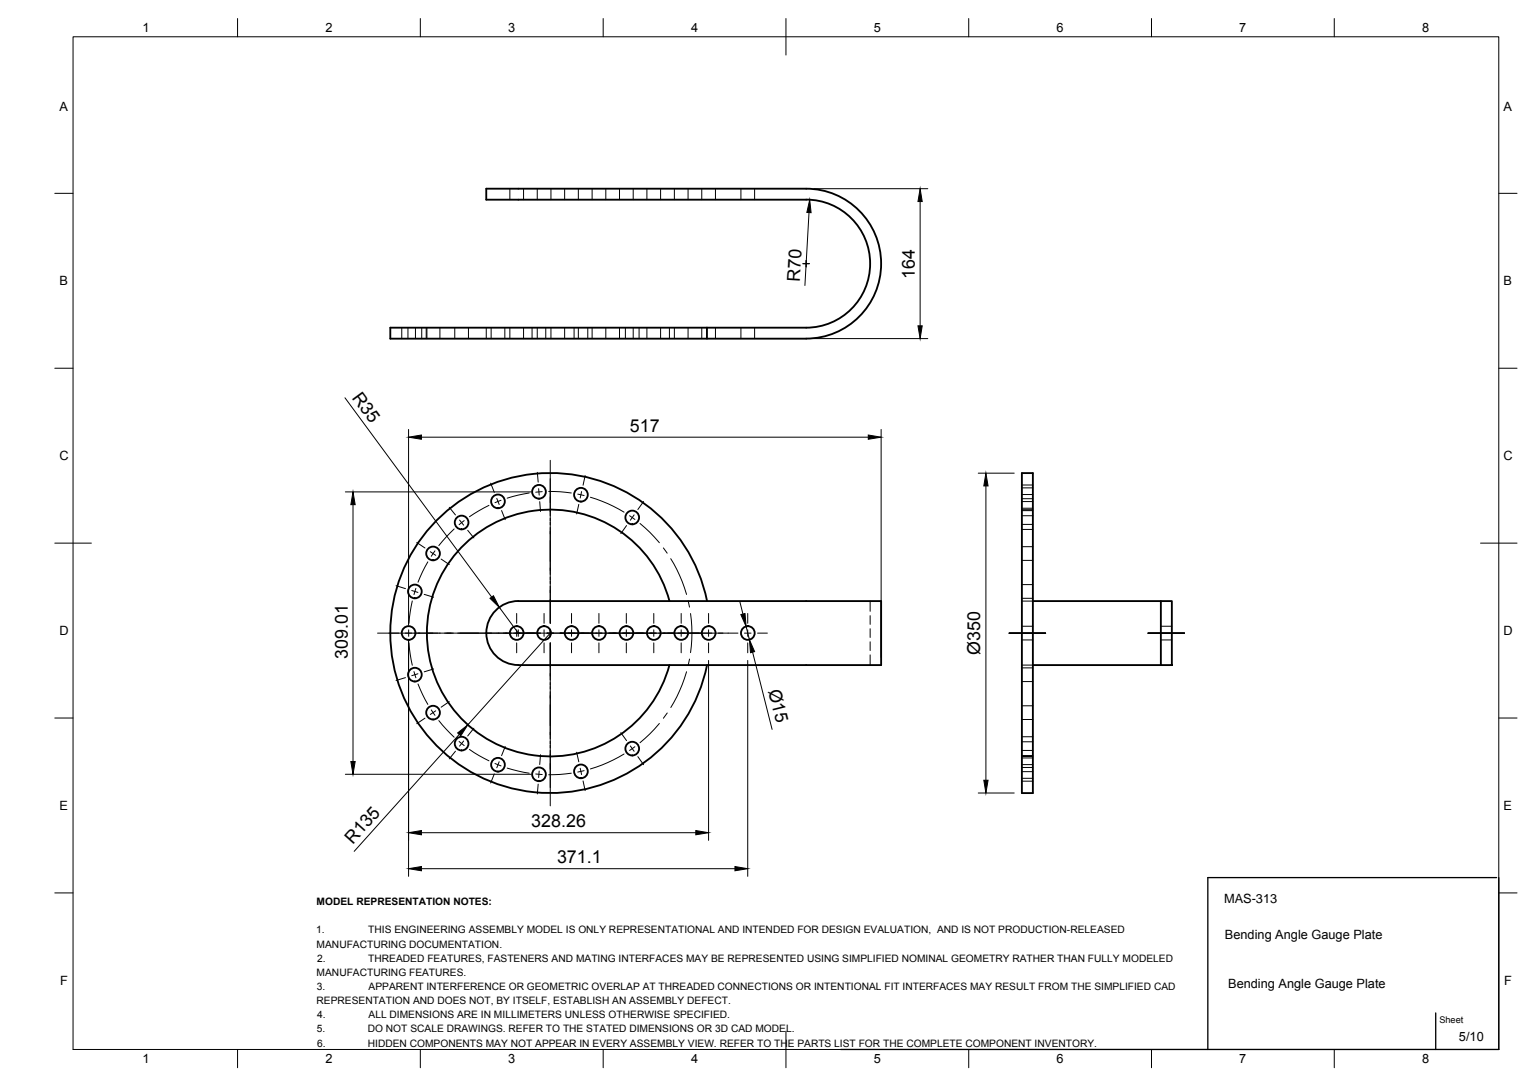
ISO-10303-21;
HEADER;
FILE_DESCRIPTION (('STEP AP214'),
    '1' );
FILE_NAME ('Bending Angle Gauge Plate.step',
    '2026-10-06T09:36:00',
    ( '' ),
    ( '' ),
    'SwSTEP 2.0',
    'SolidWorks 2025',
    '' );
FILE_SCHEMA (( 'AUTOMOTIVE_DESIGN' ));
ENDSEC;

DATA;
#1=ORIENTED_EDGE ( 'NONE', *, *, #10134, .F. ) ;
#14=EDGE_CURVE ( 'NONE', #10023, #7883, #9995, .T. ) ;
#18=CIRCLE ( 'NONE', #8899, 134.9999999999999716 ) ;
#26=DIRECTION ( 'NONE',  ( 0.000000000000000000, 0.000000000000000000, 1.000000000000000000 ) ) ;
#33=EDGE_CURVE ( 'NONE', #7221, #5849, #1766, .T. ) ;
#34=ORIENTED_EDGE ( 'NONE', *, *, #7230, .T. ) ;
#37=ORIENTED_EDGE ( 'NONE', *, *, #6606, .T. ) ;
#45=ORIENTED_EDGE ( 'NONE', *, *, #10615, .T. ) ;
#49=LINE ( 'NONE', #8712, #562 ) ;
#54=DIRECTION ( 'NONE',  ( -0.000000000000000000, 1.000000000000000000, 7.930164461608263644E-17 ) ) ;
#55=ORIENTED_EDGE ( 'NONE', *, *, #5184, .F. ) ;
#56=CARTESIAN_POINT ( 'NONE',  ( 1.561981751485805177E-12, 12.00000000000000000, 23.57864376269050410 ) ) ;
#62=FACE_BOUND ( 'NONE', #10137, .T. ) ;
#63=ORIENTED_EDGE ( 'NONE', *, *, #11154, .T. ) ;
#64=VERTEX_POINT ( 'NONE', #2451 ) ;
#74=AXIS2_PLACEMENT_3D ( 'NONE', #9091, #4403, #8176 ) ;
#75=EDGE_LOOP ( 'NONE', ( #6909, #2744, #1662, #2481 ) ) ;
#77=DIRECTION ( 'NONE',  ( 0.000000000000000000, 0.000000000000000000, 1.000000000000000000 ) ) ;
#83=VERTEX_POINT ( 'NONE', #3428 ) ;
#85=ORIENTED_EDGE ( 'NONE', *, *, #1558, .T. ) ;
#94=CYLINDRICAL_SURFACE ( 'NONE', #4643, 70.00000000000002842 ) ;
#97=AXIS2_PLACEMENT_3D ( 'NONE', #11633, #3261, #1306 ) ;
#101=ORIENTED_EDGE ( 'NONE', *, *, #4439, .T. ) ;
#110=ORIENTED_EDGE ( 'NONE', *, *, #8930, .F. ) ;
#115=DIRECTION ( 'NONE',  ( 0.000000000000000000, 1.000000000000000000, 0.000000000000000000 ) ) ;
#116=ORIENTED_EDGE ( 'NONE', *, *, #6003, .T. ) ;
#117=CYLINDRICAL_SURFACE ( 'NONE', #9034, 7.500000000000007105 ) ;
#122=ORIENTED_EDGE ( 'NONE', *, *, #10751, .T. ) ;
#123=FACE_BOUND ( 'NONE', #7167, .T. ) ;
#125=VERTEX_POINT ( 'NONE', #4313 ) ;
#131=CARTESIAN_POINT ( 'NONE',  ( -120.8820948793972434, 12.00000000000000000, -179.1989091883324363 ) ) ;
#133=VECTOR ( 'NONE', #10097, 1000.000000000000000 ) ;
#134=CARTESIAN_POINT ( 'NONE',  ( 1.387778780781445676E-14, -58.00000000000000711, 126.4213562373094959 ) ) ;
#135=ORIENTED_EDGE ( 'NONE', *, *, #8137, .F. ) ;
#148=DIRECTION ( 'NONE',  ( 0.000000000000000000, 0.000000000000000000, -1.000000000000000000 ) ) ;
#157=FACE_OUTER_BOUND ( 'NONE', #4978, .T. ) ;
#168=CYLINDRICAL_SURFACE ( 'NONE', #6692, 7.500000000000007105 ) ;
#173=ORIENTED_EDGE ( 'NONE', *, *, #11290, .T. ) ;
#175=VECTOR ( 'NONE', #6548, 1000.000000000000000 ) ;
#177=FACE_BOUND ( 'NONE', #6264, .T. ) ;
#184=ADVANCED_FACE ( 'NONE', ( #596 ), #4371, .T. ) ;
#186=CARTESIAN_POINT ( 'NONE',  ( 1.874378101782966050E-12, -6.000000000000006217, 61.07864376269051121 ) ) ;
#189=ORIENTED_EDGE ( 'NONE', *, *, #1792, .T. ) ;
#193=ORIENTED_EDGE ( 'NONE', *, *, #8592, .F. ) ;
#199=EDGE_CURVE ( 'NONE', #11915, #1856, #8826, .T. ) ;
#201=ORIENTED_EDGE ( 'NONE', *, *, #5756, .F. ) ;
#208=DIRECTION ( 'NONE',  ( -0.000000000000000000, 1.000000000000000000, 7.930164461608263644E-17 ) ) ;
#215=DIRECTION ( 'NONE',  ( -0.000000000000000000, 1.000000000000000000, 7.930164461608263644E-17 ) ) ;
#216=DIRECTION ( 'NONE',  ( 0.000000000000000000, 0.000000000000000000, 1.000000000000000000 ) ) ;
#217=ORIENTED_EDGE ( 'NONE', *, *, #11458, .T. ) ;
#224=LINE ( 'NONE', #2033, #3608 ) ;
#226=CYLINDRICAL_SURFACE ( 'NONE', #5194, 7.500000000000007105 ) ;
#231=CARTESIAN_POINT ( 'NONE',  ( 120.8820948793965186, 0.000000000000000000, -194.1989091883332890 ) ) ;
#235=EDGE_CURVE ( 'NONE', #11998, #11124, #7336, .T. ) ;
#239=CARTESIAN_POINT ( 'NONE',  ( 0.000000000000000000, 0.000000000000000000, -89.68077099980401101 ) ) ;
#241=ORIENTED_EDGE ( 'NONE', *, *, #8867, .F. ) ;
#242=CIRCLE ( 'NONE', #10114, 7.500000000000020428 ) ;
#244=CARTESIAN_POINT ( 'NONE',  ( 3.123963502971610252E-13, 12.00000000000000000, -96.42135623730949590 ) ) ;
#249=AXIS2_PLACEMENT_3D ( 'NONE', #6784, #11489, #10438 ) ;
#253=EDGE_CURVE ( 'NONE', #7231, #4288, #5520, .T. ) ;
#254=FACE_OUTER_BOUND ( 'NONE', #3985, .T. ) ;
#268=CARTESIAN_POINT ( 'NONE',  ( -35.00000000000000000, 81.99999999999998579, 190.3192290001959748 ) ) ;
#271=ADVANCED_FACE ( 'NONE', ( #9188 ), #1781, .F. ) ;
#277=ORIENTED_EDGE ( 'NONE', *, *, #5385, .T. ) ;
#278=CIRCLE ( 'NONE', #3844, 7.500000000000013323 ) ;
#281=ORIENTED_EDGE ( 'NONE', *, *, #1146, .T. ) ;
#285=CARTESIAN_POINT ( 'NONE',  ( -6.106226635438360972E-13, 0.000000000000000000, -244.6807709998039400 ) ) ;
#287=CIRCLE ( 'NONE', #5208, 7.500000000000007105 ) ;
#298=ORIENTED_EDGE ( 'NONE', *, *, #7352, .T. ) ;
#299=CARTESIAN_POINT ( 'NONE',  ( 3.123963502971610252E-13, 164.0000000000000000, -96.42135623730948168 ) ) ;
#315=ORIENTED_EDGE ( 'NONE', *, *, #3330, .T. ) ;
#319=CARTESIAN_POINT ( 'NONE',  ( 45.53315400109643463, 12.00000000000000000, -230.3419396193597208 ) ) ;
#321=EDGE_CURVE ( 'NONE', #10730, #10836, #6230, .T. ) ;
#328=EDGE_LOOP ( 'NONE', ( #135, #8709, #7075, #7838 ) ) ;
#333=DIRECTION ( 'NONE',  ( 0.000000000000000000, -1.156482317317870246E-16, 1.000000000000000000 ) ) ;
#338=VERTEX_POINT ( 'NONE', #2508 ) ;
#344=EDGE_LOOP ( 'NONE', ( #2553, #10547, #8461, #7126 ) ) ;
#348=CARTESIAN_POINT ( 'NONE',  ( 154.5043356068769071, 12.00000000000000000, -109.5666613060171670 ) ) ;
#350=CARTESIAN_POINT ( 'NONE',  ( 151.3258811035896656, 12.00000000000000000, -48.63263083939796871 ) ) ;
#356=DIRECTION ( 'NONE',  ( 0.000000000000000000, -1.000000000000000000, -7.930164461608263644E-17 ) ) ;
#362=AXIS2_PLACEMENT_3D ( 'NONE', #5126, #8886, #3258 ) ;
#367=CIRCLE ( 'NONE', #4729, 7.500000000000007105 ) ;
#371=CIRCLE ( 'NONE', #8725, 7.500000000000007105 ) ;
#383=EDGE_LOOP ( 'NONE', ( #2203, #8907 ) ) ;
#384=CARTESIAN_POINT ( 'NONE',  ( -151.3258811035894098, 12.00000000000000000, -48.63263083939678921 ) ) ;
#386=ORIENTED_EDGE ( 'NONE', *, *, #9875, .T. ) ;
#394=CYLINDRICAL_SURFACE ( 'NONE', #10869, 134.9999999999999716 ) ;
#403=EDGE_CURVE ( 'NONE', #4980, #6173, #8091, .T. ) ;
#404=FACE_BOUND ( 'NONE', #5340, .T. ) ;
#409=CARTESIAN_POINT ( 'NONE',  ( 1.874378101782966050E-12, 152.0000000000000000, 53.57864376269051832 ) ) ;
#411=DIRECTION ( 'NONE',  ( -0.000000000000000000, -1.000000000000000000, -0.000000000000000000 ) ) ;
#420=DIRECTION ( 'NONE',  ( -0.000000000000000000, 1.000000000000000000, 0.000000000000000000 ) ) ;
#421=DIRECTION ( 'NONE',  ( 0.000000000000000000, -1.189524669241239115E-16, 1.000000000000000000 ) ) ;
#422=LINE ( 'NONE', #11515, #6475 ) ;
#424=EDGE_LOOP ( 'NONE', ( #6274, #101, #7246, #3774 ) ) ;
#428=ORIENTED_EDGE ( 'NONE', *, *, #8066, .T. ) ;
#431=DIRECTION ( 'NONE',  ( 0.000000000000000000, 0.000000000000000000, 1.000000000000000000 ) ) ;
#435=ORIENTED_EDGE ( 'NONE', *, *, #33, .T. ) ;
#444=CARTESIAN_POINT ( 'NONE',  ( -35.00000000000000000, 12.00000000000000000, 81.78351099501843180 ) ) ;
#450=DIRECTION ( 'NONE',  ( 0.000000000000000000, 0.000000000000000000, 1.000000000000000000 ) ) ;
#452=ORIENTED_EDGE ( 'NONE', *, *, #4862, .T. ) ;
#455=DIRECTION ( 'NONE',  ( 0.000000000000000000, -1.000000000000000000, -7.930164461608263644E-17 ) ) ;
#458=DIRECTION ( 'NONE',  ( -0.000000000000000000, -1.000000000000000000, -0.000000000000000000 ) ) ;
#461=AXIS2_PLACEMENT_3D ( 'NONE', #12105, #7277, #8143 ) ;
#463=AXIS2_PLACEMENT_3D ( 'NONE', #244, #1196, #4029 ) ;
#468=EDGE_CURVE ( 'NONE', #6717, #8440, #6310, .T. ) ;
#473=CARTESIAN_POINT ( 'NONE',  ( 1.387778780781445676E-14, 163.9999999999999716, 126.4213562373094959 ) ) ;
#474=CIRCLE ( 'NONE', #2458, 7.500000000000007105 ) ;
#482=VECTOR ( 'NONE', #7675, 1000.000000000000000 ) ;
#484=FACE_BOUND ( 'NONE', #2793, .T. ) ;
#492=ADVANCED_FACE ( 'NONE', ( #8638 ), #1164, .F. ) ;
#498=ORIENTED_EDGE ( 'NONE', *, *, #8039, .T. ) ;
#502=VERTEX_POINT ( 'NONE', #6093 ) ;
#508=LINE ( 'NONE', #9976, #3240 ) ;
#519=DIRECTION ( 'NONE',  ( -0.000000000000000000, 1.000000000000000000, 7.930164461608263644E-17 ) ) ;
#525=CARTESIAN_POINT ( 'NONE',  ( 9.381075359908434252E-13, 152.0000000000000000, -43.92135623730948879 ) ) ;
#533=FACE_BOUND ( 'NONE', #4273, .T. ) ;
#540=DIRECTION ( 'NONE',  ( 0.000000000000000000, -1.000000000000000000, -7.930164461608263644E-17 ) ) ;
#543=CARTESIAN_POINT ( 'NONE',  ( 3.133148353965215262E-13, 164.0000000000000000, -103.9213562373094817 ) ) ;
#544=EDGE_CURVE ( 'NONE', #10381, #12119, #6034, .T. ) ;
#550=DIRECTION ( 'NONE',  ( 0.000000000000000000, -1.000000000000000000, -7.930164461608263644E-17 ) ) ;
#554=CARTESIAN_POINT ( 'NONE',  ( 151.3258811035896656, 12.00000000000000000, -48.63263083939796871 ) ) ;
#560=LINE ( 'NONE', #4380, #7867 ) ;
#562=VECTOR ( 'NONE', #6726, 1000.000000000000000 ) ;
#564=EDGE_CURVE ( 'NONE', #918, #10860, #2578, .T. ) ;
#566=EDGE_CURVE ( 'NONE', #8781, #8293, #8892, .T. ) ;
#571=AXIS2_PLACEMENT_3D ( 'NONE', #8163, #1546, #11066 ) ;
#572=DIRECTION ( 'NONE',  ( 0.000000000000000000, 0.000000000000000000, 1.000000000000000000 ) ) ;
#584=CARTESIAN_POINT ( 'NONE',  ( -35.00000000000000000, 2.012279232133096230E-14, -124.6807709998040110 ) ) ;
#596=FACE_OUTER_BOUND ( 'NONE', #11058, .T. ) ;
#599=CARTESIAN_POINT ( 'NONE',  ( 1.561981751485805177E-12, 163.9999999999999716, 23.57864376269051832 ) ) ;
#601=EDGE_LOOP ( 'NONE', ( #8052, #9724 ) ) ;
#604=DIRECTION ( 'NONE',  ( 0.000000000000000000, 0.000000000000000000, 1.000000000000000000 ) ) ;
#605=CARTESIAN_POINT ( 'NONE',  ( 1.562900236585165577E-12, 152.0000000000000000, 16.07864376269051121 ) ) ;
#613=FACE_BOUND ( 'NONE', #10660, .T. ) ;
#615=DIRECTION ( 'NONE',  ( 0.000000000000000000, 0.000000000000000000, -1.000000000000000000 ) ) ;
#621=CIRCLE ( 'NONE', #9099, 7.500000000000007105 ) ;
#622=ADVANCED_FACE ( 'NONE', ( #9861 ), #394, .F. ) ;
#626=EDGE_LOOP ( 'NONE', ( #6311, #2844 ) ) ;
#631=ORIENTED_EDGE ( 'NONE', *, *, #733, .T. ) ;
#640=DIRECTION ( 'NONE',  ( 0.000000000000000000, 1.000000000000000000, 0.000000000000000000 ) ) ;
#645=DIRECTION ( 'NONE',  ( 0.000000000000000000, 0.000000000000000000, 1.000000000000000000 ) ) ;
#647=VERTEX_POINT ( 'NONE', #1446 ) ;
#650=EDGE_LOOP ( 'NONE', ( #11783, #7128, #2797, #3359 ) ) ;
#656=DIRECTION ( 'NONE',  ( -0.000000000000000000, -1.000000000000000000, -0.000000000000000000 ) ) ;
#660=CARTESIAN_POINT ( 'NONE',  ( -126.4213562373094959, 0.000000000000000000, 7.500000000000036415 ) ) ;
#663=CARTESIAN_POINT ( 'NONE',  ( 1.874378101782966050E-12, 163.9999999999999716, 53.57864376269051832 ) ) ;
#670=FACE_OUTER_BOUND ( 'NONE', #424, .T. ) ;
#671=DIRECTION ( 'NONE',  ( 0.000000000000000000, 0.000000000000000000, 1.000000000000000000 ) ) ;
#672=AXIS2_PLACEMENT_3D ( 'NONE', #2277, #7090, #6167 ) ;
#675=ORIENTED_EDGE ( 'NONE', *, *, #9229, .F. ) ;
#682=LINE ( 'NONE', #10016, #4219 ) ;
#685=ORIENTED_EDGE ( 'NONE', *, *, #5256, .T. ) ;
#687=ORIENTED_EDGE ( 'NONE', *, *, #9653, .F. ) ;
#688=DIRECTION ( 'NONE',  ( 0.000000000000000000, 0.000000000000000000, -1.000000000000000000 ) ) ;
#693=CIRCLE ( 'NONE', #7604, 70.00000000000002842 ) ;
#694=VERTEX_POINT ( 'NONE', #2685 ) ;
#701=EDGE_LOOP ( 'NONE', ( #6324, #2440, #6315, #11484 ) ) ;
#707=DIRECTION ( 'NONE',  ( 0.000000000000000000, -1.000000000000000000, -7.930164461608263644E-17 ) ) ;
#720=VECTOR ( 'NONE', #6752, 1000.000000000000000 ) ;
#722=DIRECTION ( 'NONE',  ( 0.000000000000000000, 0.000000000000000000, 1.000000000000000000 ) ) ;
#723=DIRECTION ( 'NONE',  ( -0.000000000000000000, 1.000000000000000000, 7.930164461608263644E-17 ) ) ;
#725=VERTEX_POINT ( 'NONE', #9236 ) ;
#731=CARTESIAN_POINT ( 'NONE',  ( 1.479627290717497352E-14, 11.99999999999999645, 118.9213562373094817 ) ) ;
#733=EDGE_CURVE ( 'NONE', #10254, #9573, #1405, .T. ) ;
#734=CARTESIAN_POINT ( 'NONE',  ( 45.53315400109643463, 0.000000000000000000, -237.8419396193597208 ) ) ;
#736=CARTESIAN_POINT ( 'NONE',  ( 154.5043356068769071, 12.00000000000000000, -102.0666613060171386 ) ) ;
#739=VERTEX_POINT ( 'NONE', #4550 ) ;
#748=ORIENTED_EDGE ( 'NONE', *, *, #9825, .T. ) ;
#749=DIRECTION ( 'NONE',  ( 0.000000000000000000, 0.000000000000000000, -1.000000000000000000 ) ) ;
#753=EDGE_LOOP ( 'NONE', ( #7953, #4531, #9259, #7729, #4093, #3852, #8510, #4536, #872, #2326 ) ) ;
#762=DIRECTION ( 'NONE',  ( 0.000000000000000000, 1.000000000000000000, 0.000000000000000000 ) ) ;
#763=DIRECTION ( 'NONE',  ( -0.000000000000000000, -1.000000000000000000, -0.000000000000000000 ) ) ;
#766=DIRECTION ( 'NONE',  ( 0.000000000000000000, 0.000000000000000000, -1.000000000000000000 ) ) ;
#777=CARTESIAN_POINT ( 'NONE',  ( 0.000000000000000000, 12.00000000000000000, -89.68077099980401101 ) ) ;
#789=EDGE_CURVE ( 'NONE', #11268, #694, #18, .T. ) ;
#790=DIRECTION ( 'NONE',  ( -0.000000000000000000, 1.000000000000000000, 7.930164461608263644E-17 ) ) ;
#796=DIRECTION ( 'NONE',  ( 0.000000000000000000, 1.000000000000000000, 0.000000000000000000 ) ) ;
#797=ORIENTED_EDGE ( 'NONE', *, *, #3584, .F. ) ;
#798=EDGE_LOOP ( 'NONE', ( #9828, #5326 ) ) ;
#799=DIRECTION ( 'NONE',  ( 0.000000000000000000, 1.000000000000000000, 0.000000000000000000 ) ) ;
#802=ORIENTED_EDGE ( 'NONE', *, *, #5618, .F. ) ;
#806=DIRECTION ( 'NONE',  ( 0.000000000000000000, 0.000000000000000000, -1.000000000000000000 ) ) ;
#810=ORIENTED_EDGE ( 'NONE', *, *, #11144, .T. ) ;
#812=CARTESIAN_POINT ( 'NONE',  ( 1.561981751485805177E-12, 163.9999999999999716, 31.07864376269052542 ) ) ;
#819=CYLINDRICAL_SURFACE ( 'NONE', #3637, 7.500000000000007105 ) ;
#827=ORIENTED_EDGE ( 'NONE', *, *, #9947, .T. ) ;
#832=ORIENTED_EDGE ( 'NONE', *, *, #4675, .F. ) ;
#834=DIRECTION ( 'NONE',  ( 0.000000000000000000, 0.000000000000000000, 1.000000000000000000 ) ) ;
#837=ORIENTED_EDGE ( 'NONE', *, *, #12209, .F. ) ;
#838=CARTESIAN_POINT ( 'NONE',  ( 154.5043356068769071, 12.00000000000000000, -102.0666613060171386 ) ) ;
#841=CARTESIAN_POINT ( 'NONE',  ( 35.00000000000000000, 82.00000000000071054, -124.6807709998040394 ) ) ;
#848=AXIS2_PLACEMENT_3D ( 'NONE', #5293, #9070, #604 ) ;
#852=ORIENTED_EDGE ( 'NONE', *, *, #4369, .F. ) ;
#854=DIRECTION ( 'NONE',  ( -0.000000000000000000, 1.000000000000000000, 7.930164461608263644E-17 ) ) ;
#871=AXIS2_PLACEMENT_3D ( 'NONE', #2824, #2567, #2628 ) ;
#872=ORIENTED_EDGE ( 'NONE', *, *, #898, .T. ) ;
#875=CARTESIAN_POINT ( 'NONE',  ( -154.5043356068770493, 12.00000000000000000, -94.56666130601601594 ) ) ;
#879=DIRECTION ( 'NONE',  ( 0.000000000000000000, 0.000000000000000000, 1.000000000000000000 ) ) ;
#881=CARTESIAN_POINT ( 'NONE',  ( 2.186774452080127126E-12, 0.000000000000000000, 83.57864376269050410 ) ) ;
#889=ORIENTED_EDGE ( 'NONE', *, *, #11610, .F. ) ;
#890=EDGE_LOOP ( 'NONE', ( #10634, #2205 ) ) ;
#891=AXIS2_PLACEMENT_3D ( 'NONE', #6379, #6445, #10149 ) ;
#892=AXIS2_PLACEMENT_3D ( 'NONE', #10290, #12162, #2817 ) ;
#893=DIRECTION ( 'NONE',  ( 0.000000000000000000, 1.000000000000000000, 0.000000000000000000 ) ) ;
#895=AXIS2_PLACEMENT_3D ( 'NONE', #268, #10484, #4853 ) ;
#897=EDGE_LOOP ( 'NONE', ( #5030, #10337, #10470, #5661 ) ) ;
#898=EDGE_CURVE ( 'NONE', #2093, #11305, #6146, .T. ) ;
#900=CARTESIAN_POINT ( 'NONE',  ( 0.000000000000000000, 152.0000000000000284, -126.4213562373094959 ) ) ;
#901=DIRECTION ( 'NONE',  ( 0.000000000000000000, 0.000000000000000000, 1.000000000000000000 ) ) ;
#906=CIRCLE ( 'NONE', #10557, 70.00000000000002842 ) ;
#907=DIRECTION ( 'NONE',  ( 0.000000000000000000, 0.000000000000000000, 1.000000000000000000 ) ) ;
#908=DIRECTION ( 'NONE',  ( 0.000000000000000000, -1.189524669241239115E-16, 1.000000000000000000 ) ) ;
#918=VERTEX_POINT ( 'NONE', #2812 ) ;
#920=CARTESIAN_POINT ( 'NONE',  ( 1.249585401188644101E-12, 0.000000000000000000, 1.078643762690513874 ) ) ;
#930=CARTESIAN_POINT ( 'NONE',  ( 1.874378101782966050E-12, -6.000000000000005329, 53.57864376269050410 ) ) ;
#931=VERTEX_POINT ( 'NONE', #4901 ) ;
#933=CARTESIAN_POINT ( 'NONE',  ( 35.00000000000000000, 2.428612866367529932E-14, -159.6807709998040252 ) ) ;
#939=DIRECTION ( 'NONE',  ( -0.000000000000000000, -1.000000000000000000, -0.000000000000000000 ) ) ;
#944=EDGE_CURVE ( 'NONE', #3591, #6687, #10892, .T. ) ;
#954=CARTESIAN_POINT ( 'NONE',  ( 87.04832655144112152, 12.00000000000000000, -225.4289243767383368 ) ) ;
#956=DIRECTION ( 'NONE',  ( 0.000000000000000000, 0.000000000000000000, 1.000000000000000000 ) ) ;
#961=DIRECTION ( 'NONE',  ( 0.000000000000000000, 1.000000000000000000, 0.000000000000000000 ) ) ;
#974=FACE_OUTER_BOUND ( 'NONE', #10045, .T. ) ;
#984=ORIENTED_EDGE ( 'NONE', *, *, #5781, .T. ) ;
#986=CARTESIAN_POINT ( 'NONE',  ( -35.00000000000000000, 81.99999999999998579, 190.3192290001959748 ) ) ;
#987=DIRECTION ( 'NONE',  ( -0.000000000000000000, 1.000000000000000000, 7.930164461608263644E-17 ) ) ;
#992=CARTESIAN_POINT ( 'NONE',  ( 2.187692937179487324E-12, 0.000000000000000000, 76.07864376269048989 ) ) ;
#997=CARTESIAN_POINT ( 'NONE',  ( 6.247927005943220505E-13, -6.000000000000005329, -66.42135623730949590 ) ) ;
#998=ORIENTED_EDGE ( 'NONE', *, *, #33, .F. ) ;
#1000=VERTEX_POINT ( 'NONE', #10591 ) ;
#1003=FACE_BOUND ( 'NONE', #3356, .T. ) ;
#1004=ORIENTED_EDGE ( 'NONE', *, *, #1417, .F. ) ;
#1005=ORIENTED_EDGE ( 'NONE', *, *, #566, .F. ) ;
#1020=CARTESIAN_POINT ( 'NONE',  ( 0.000000000000000000, 12.00000000000000000, -224.6807709998039968 ) ) ;
#1024=DIRECTION ( 'NONE',  ( 0.000000000000000000, 0.000000000000000000, 1.000000000000000000 ) ) ;
#1042=CARTESIAN_POINT ( 'NONE',  ( 120.8820948793965186, 0.000000000000000000, -186.6989091883332890 ) ) ;
#1049=ADVANCED_FACE ( 'NONE', ( #9076 ), #5081, .F. ) ;
#1065=DIRECTION ( 'NONE',  ( -0.000000000000000000, 1.000000000000000000, 7.930164461608263644E-17 ) ) ;
#1068=FACE_BOUND ( 'NONE', #9922, .T. ) ;
#1072=LINE ( 'NONE', #8442, #4255 ) ;
#1086=AXIS2_PLACEMENT_3D ( 'NONE', #9773, #2360, #1314 ) ;
#1087=LINE ( 'NONE', #2128, #5843 ) ;
#1096=ORIENTED_EDGE ( 'NONE', *, *, #2654, .F. ) ;
#1098=ADVANCED_FACE ( 'NONE', ( #11061 ), #7814, .F. ) ;
#1100=CARTESIAN_POINT ( 'NONE',  ( 35.00000000000000000, 152.0000000000000000, 190.3192290001959748 ) ) ;
#1109=ORIENTED_EDGE ( 'NONE', *, *, #2855, .T. ) ;
#1117=DIRECTION ( 'NONE',  ( 0.000000000000000000, 0.000000000000000000, -1.000000000000000000 ) ) ;
#1118=CARTESIAN_POINT ( 'NONE',  ( -35.00000000000000000, 0.000000000000000000, 40.70327710424895429 ) ) ;
#1122=CARTESIAN_POINT ( 'NONE',  ( 1.249585401188644101E-12, 12.00000000000000000, -6.421356237309494119 ) ) ;
#1129=ORIENTED_EDGE ( 'NONE', *, *, #199, .F. ) ;
#1131=EDGE_CURVE ( 'NONE', #4910, #2378, #6110, .T. ) ;
#1135=LINE ( 'NONE', #8726, #2644 ) ;
#1143=EDGE_LOOP ( 'NONE', ( #4148, #428, #10091, #5318 ) ) ;
#1145=CARTESIAN_POINT ( 'NONE',  ( 1.249585401188644101E-12, -6.000000000000005329, -6.421356237309495008 ) ) ;
#1146=EDGE_CURVE ( 'NONE', #5183, #3163, #12052, .T. ) ;
#1153=CARTESIAN_POINT ( 'NONE',  ( 1.874378101782966050E-12, 0.000000000000000000, 53.57864376269050410 ) ) ;
#1164=CYLINDRICAL_SURFACE ( 'NONE', #4575, 7.500000000000007105 ) ;
#1165=CIRCLE ( 'NONE', #1752, 7.500000000000007105 ) ;
#1173=DIRECTION ( 'NONE',  ( 0.000000000000000000, 0.000000000000000000, 1.000000000000000000 ) ) ;
#1174=VECTOR ( 'NONE', #7048, 1000.000000000000000 ) ;
#1176=ORIENTED_EDGE ( 'NONE', *, *, #10134, .T. ) ;
#1179=DIRECTION ( 'NONE',  ( 0.000000000000000000, 1.000000000000000000, 0.000000000000000000 ) ) ;
#1180=DIRECTION ( 'NONE',  ( 0.000000000000000000, 1.000000000000000000, 0.000000000000000000 ) ) ;
#1181=CLOSED_SHELL ( 'NONE', ( #2542, #11758, #7956, #2235, #4789, #7074, #2002, #8291, #11705, #2213, #9575, #4708, #4730, #9794, #7659, #7989, #5207, #11669, #184, #11079, #9868, #10769, #3546, #2306, #7612, #3183, #8173, #8650, #6552, #8788, #4998, #11606, #9913, #7159, #4622, #1812, #9562, #9491, #1866, #10155, #622, #1425, #5384, #10291, #6067, #7120, #1098, #2092, #9108, #8853, #4168, #7313, #4187, #12137, #1049, #3430, #8221, #5456, #7889, #10174, #11655, #10828, #5327, #3009, #7053, #5388, #11450, #11950, #1268, #11478, #6978, #8435, #4881, #271, #4641, #10024, #8378, #2223, #6168, #5705, #5012, #492, #7320, #11734 ) ) ;
#1183=DIRECTION ( 'NONE',  ( -0.000000000000000000, 1.000000000000000000, -0.000000000000000000 ) ) ;
#1191=FACE_BOUND ( 'NONE', #5209, .T. ) ;
#1196=DIRECTION ( 'NONE',  ( 0.000000000000000000, 1.000000000000000000, 0.000000000000000000 ) ) ;
#1199=CARTESIAN_POINT ( 'NONE',  ( -151.3258811035894098, 0.000000000000000000, -63.63263083939681053 ) ) ;
#1201=EDGE_CURVE ( 'NONE', #1440, #4090, #3564, .T. ) ;
#1213=ORIENTED_EDGE ( 'NONE', *, *, #10066, .T. ) ;
#1216=DIRECTION ( 'NONE',  ( -1.000000000000000000, -0.000000000000000000, -0.000000000000000000 ) ) ;
#1221=CARTESIAN_POINT ( 'NONE',  ( 35.00000000000000000, 11.99999999999998046, 190.3192290001959748 ) ) ;
#1223=ORIENTED_EDGE ( 'NONE', *, *, #8229, .T. ) ;
#1225=ORIENTED_EDGE ( 'NONE', *, *, #8680, .T. ) ;
#1230=CYLINDRICAL_SURFACE ( 'NONE', #10295, 7.500000000000007105 ) ;
#1234=DIRECTION ( 'NONE',  ( 0.000000000000000000, 0.000000000000000000, 1.000000000000000000 ) ) ;
#1239=EDGE_LOOP ( 'NONE', ( #9550, #3658, #281, #8822 ) ) ;
#1243=CARTESIAN_POINT ( 'NONE',  ( 144.0488662551573782, 12.00000000000000000, -146.9077238332702109 ) ) ;
#1247=ORIENTED_EDGE ( 'NONE', *, *, #5033, .F. ) ;
#1248=ORIENTED_EDGE ( 'NONE', *, *, #3362, .F. ) ;
#1254=AXIS2_PLACEMENT_3D ( 'NONE', #6991, #1846, #12108 ) ;
#1256=ORIENTED_EDGE ( 'NONE', *, *, #8467, .T. ) ;
#1257=CIRCLE ( 'NONE', #2842, 7.500000000000007105 ) ;
#1264=DIRECTION ( 'NONE',  ( 0.000000000000000000, 0.000000000000000000, -1.000000000000000000 ) ) ;
#1265=ORIENTED_EDGE ( 'NONE', *, *, #14, .F. ) ;
#1267=ORIENTED_EDGE ( 'NONE', *, *, #1417, .T. ) ;
#1268=ADVANCED_FACE ( 'NONE', ( #6489 ), #1795, .F. ) ;
#1269=EDGE_CURVE ( 'NONE', #1000, #4907, #9397, .T. ) ;
#1271=ORIENTED_EDGE ( 'NONE', *, *, #2172, .T. ) ;
#1273=AXIS2_PLACEMENT_3D ( 'NONE', #4077, #10676, #6045 ) ;
#1280=CARTESIAN_POINT ( 'NONE',  ( 0.000000000000000000, 12.00000000000000000, -89.68077099980401101 ) ) ;
#1281=VECTOR ( 'NONE', #4648, 1000.000000000000000 ) ;
#1285=CYLINDRICAL_SURFACE ( 'NONE', #2633, 7.500000000000007994 ) ;
#1286=ORIENTED_EDGE ( 'NONE', *, *, #3121, .T. ) ;
#1290=LINE ( 'NONE', #9686, #7073 ) ;
#1291=VECTOR ( 'NONE', #5339, 1000.000000000000000 ) ;
#1292=DIRECTION ( 'NONE',  ( -0.000000000000000000, 1.000000000000000000, 7.930164461608263644E-17 ) ) ;
#1297=DIRECTION ( 'NONE',  ( -0.000000000000000000, -1.000000000000000000, -0.000000000000000000 ) ) ;
#1301=ORIENTED_EDGE ( 'NONE', *, *, #8271, .T. ) ;
#1304=DIRECTION ( 'NONE',  ( 0.000000000000000000, -1.156482317317870246E-16, 1.000000000000000000 ) ) ;
#1306=DIRECTION ( 'NONE',  ( 0.000000000000000000, 0.000000000000000000, 1.000000000000000000 ) ) ;
#1312=EDGE_CURVE ( 'NONE', #4553, #11886, #371, .T. ) ;
#1314=DIRECTION ( 'NONE',  ( 0.000000000000000000, 0.000000000000000000, 1.000000000000000000 ) ) ;
#1317=AXIS2_PLACEMENT_3D ( 'NONE', #7563, #10403, #1944 ) ;
#1319=EDGE_CURVE ( 'NONE', #6750, #5569, #8539, .T. ) ;
#1330=VERTEX_POINT ( 'NONE', #9693 ) ;
#1333=AXIS2_PLACEMENT_3D ( 'NONE', #6232, #6112, #9997 ) ;
#1335=AXIS2_PLACEMENT_3D ( 'NONE', #4486, #3599, #5334 ) ;
#1339=ORIENTED_EDGE ( 'NONE', *, *, #10551, .F. ) ;
#1340=CARTESIAN_POINT ( 'NONE',  ( 1.249585401188644101E-12, -6.000000000000005329, -6.421356237309495008 ) ) ;
#1360=AXIS2_PLACEMENT_3D ( 'NONE', #7115, #7050, #5314 ) ;
#1363=CARTESIAN_POINT ( 'NONE',  ( 35.00000000000000000, 81.99999999999998579, 190.3192290001959748 ) ) ;
#1376=ORIENTED_EDGE ( 'NONE', *, *, #3295, .T. ) ;
#1382=DIRECTION ( 'NONE',  ( -0.000000000000000000, -1.000000000000000000, -0.000000000000000000 ) ) ;
#1386=CARTESIAN_POINT ( 'NONE',  ( 0.000000000000000000, 0.000000000000000000, -89.68077099980401101 ) ) ;
#1389=CARTESIAN_POINT ( 'NONE',  ( 87.04832655144112152, 0.000000000000000000, -210.4289243767383368 ) ) ;
#1392=DIRECTION ( 'NONE',  ( -0.000000000000000000, -1.000000000000000000, -0.000000000000000000 ) ) ;
#1394=CYLINDRICAL_SURFACE ( 'NONE', #8761, 7.500000000000007105 ) ;
#1396=VERTEX_POINT ( 'NONE', #9514 ) ;
#1401=CYLINDRICAL_SURFACE ( 'NONE', #1751, 7.500000000000007105 ) ;
#1404=DIRECTION ( 'NONE',  ( -1.000000000000000000, -0.000000000000000000, 0.000000000000000000 ) ) ;
#1405=CIRCLE ( 'NONE', #2989, 7.500000000000007105 ) ;
#1409=FACE_BOUND ( 'NONE', #5480, .T. ) ;
#1417=EDGE_CURVE ( 'NONE', #1330, #4052, #621, .T. ) ;
#1422=DIRECTION ( 'NONE',  ( 0.000000000000000000, 0.000000000000000000, 1.000000000000000000 ) ) ;
#1424=ORIENTED_EDGE ( 'NONE', *, *, #8431, .F. ) ;
#1425=ADVANCED_FACE ( 'NONE', ( #9933, #4261, #1468, #6971, #3253, #2278, #1409, #10985, #5227, #4373, #4315, #404, #6046, #3368, #533, #7031, #8089, #8027, #11796, #9814, #8144, #8999, #2511, #7155, #10801, #10922 ), #2453, .T. ) ;
#1429=LINE ( 'NONE', #6874, #9250 ) ;
#1431=CARTESIAN_POINT ( 'NONE',  ( -6.106226635438360972E-13, 12.00000000000000000, -244.6807709998039400 ) ) ;
#1433=ORIENTED_EDGE ( 'NONE', *, *, #11520, .T. ) ;
#1440=VERTEX_POINT ( 'NONE', #2340 ) ;
#1446=CARTESIAN_POINT ( 'NONE',  ( 144.0488662551573782, 12.00000000000000000, -154.4077238332702393 ) ) ;
#1452=EDGE_CURVE ( 'NONE', #8333, #2076, #1529, .T. ) ;
#1454=CARTESIAN_POINT ( 'NONE',  ( 126.4213562373094959, 12.00000000000000000, -7.500000000000020428 ) ) ;
#1455=VERTEX_POINT ( 'NONE', #8934 ) ;
#1457=EDGE_CURVE ( 'NONE', #3163, #7119, #2798, .T. ) ;
#1458=CARTESIAN_POINT ( 'NONE',  ( 1.387778780781445676E-14, 152.0000000000000284, 133.9213562373095101 ) ) ;
#1462=EDGE_CURVE ( 'NONE', #11305, #5102, #6287, .T. ) ;
#1468=FACE_BOUND ( 'NONE', #7001, .T. ) ;
#1469=LINE ( 'NONE', #4374, #2539 ) ;
#1483=ORIENTED_EDGE ( 'NONE', *, *, #2370, .F. ) ;
#1486=VECTOR ( 'NONE', #10909, 1000.000000000000000 ) ;
#1487=CARTESIAN_POINT ( 'NONE',  ( 0.000000000000000000, -58.00000000000000711, -118.9213562373094817 ) ) ;
#1490=DIRECTION ( 'NONE',  ( 0.000000000000000000, 1.000000000000000000, 0.000000000000000000 ) ) ;
#1493=VERTEX_POINT ( 'NONE', #7121 ) ;
#1503=ORIENTED_EDGE ( 'NONE', *, *, #12036, .F. ) ;
#1504=AXIS2_PLACEMENT_3D ( 'NONE', #5650, #9422, #8504 ) ;
#1506=CARTESIAN_POINT ( 'NONE',  ( -151.3258811035894098, 12.00000000000000000, -63.63263083939681053 ) ) ;
#1507=FACE_OUTER_BOUND ( 'NONE', #10961, .T. ) ;
#1508=AXIS2_PLACEMENT_3D ( 'NONE', #4557, #2694, #9310 ) ;
#1510=DIRECTION ( 'NONE',  ( 0.000000000000000000, 0.000000000000000000, 1.000000000000000000 ) ) ;
#1517=CARTESIAN_POINT ( 'NONE',  ( -35.00000000000000000, 12.00000000000001954, -124.6807709998040110 ) ) ;
#1522=DIRECTION ( 'NONE',  ( -0.000000000000000000, 1.000000000000000000, 7.930164461608263644E-17 ) ) ;
#1525=AXIS2_PLACEMENT_3D ( 'NONE', #4084, #10684, #7854 ) ;
#1529=LINE ( 'NONE', #5287, #5068 ) ;
#1536=DIRECTION ( 'NONE',  ( 0.000000000000000000, -1.156482317317870246E-16, 1.000000000000000000 ) ) ;
#1538=CIRCLE ( 'NONE', #12208, 7.500000000000007105 ) ;
#1539=CYLINDRICAL_SURFACE ( 'NONE', #8352, 7.500000000000007105 ) ;
#1544=VECTOR ( 'NONE', #7610, 1000.000000000000000 ) ;
#1545=EDGE_CURVE ( 'NONE', #8717, #4751, #224, .T. ) ;
#1546=DIRECTION ( 'NONE',  ( -0.000000000000000000, 1.000000000000000000, 0.000000000000000000 ) ) ;
#1548=DIRECTION ( 'NONE',  ( -0.000000000000000000, 1.000000000000000000, -0.000000000000000000 ) ) ;
#1554=ORIENTED_EDGE ( 'NONE', *, *, #9478, .T. ) ;
#1558=EDGE_CURVE ( 'NONE', #11124, #5668, #5379, .T. ) ;
#1559=ORIENTED_EDGE ( 'NONE', *, *, #7371, .T. ) ;
#1563=AXIS2_PLACEMENT_3D ( 'NONE', #10918, #10856, #11737 ) ;
#1564=ORIENTED_EDGE ( 'NONE', *, *, #5371, .T. ) ;
#1576=EDGE_LOOP ( 'NONE', ( #4875, #298 ) ) ;
#1578=LINE ( 'NONE', #1706, #1486 ) ;
#1579=ORIENTED_EDGE ( 'NONE', *, *, #2760, .T. ) ;
#1583=CARTESIAN_POINT ( 'NONE',  ( -6.106226635438360972E-13, 0.000000000000000000, -252.1807709998039115 ) ) ;
#1585=DIRECTION ( 'NONE',  ( 0.000000000000000000, 0.000000000000000000, 1.000000000000000000 ) ) ;
#1586=DIRECTION ( 'NONE',  ( -1.000000000000000000, -0.000000000000000000, -0.000000000000000000 ) ) ;
#1587=DIRECTION ( 'NONE',  ( 0.000000000000000000, -1.156482317317870246E-16, 1.000000000000000000 ) ) ;
#1594=LINE ( 'NONE', #8942, #5885 ) ;
#1595=CARTESIAN_POINT ( 'NONE',  ( 0.000000000000000000, -58.00000000000000711, -126.4213562373094959 ) ) ;
#1603=CARTESIAN_POINT ( 'NONE',  ( 1.875296586882326249E-12, 0.000000000000000000, 46.07864376269049700 ) ) ;
#1613=EDGE_CURVE ( 'NONE', #4601, #7504, #3029, .T. ) ;
#1614=DIRECTION ( 'NONE',  ( -0.000000000000000000, 1.000000000000000000, 7.930164461608263644E-17 ) ) ;
#1618=VECTOR ( 'NONE', #6678, 1000.000000000000000 ) ;
#1619=EDGE_CURVE ( 'NONE', #9863, #5323, #9346, .T. ) ;
#1621=CARTESIAN_POINT ( 'NONE',  ( -154.5043356068770493, 12.00000000000000000, -102.0666613060160302 ) ) ;
#1631=CARTESIAN_POINT ( 'NONE',  ( 1.561981751485805177E-12, 152.0000000000000000, 23.57864376269051832 ) ) ;
#1636=ORIENTED_EDGE ( 'NONE', *, *, #1312, .F. ) ;
#1639=CARTESIAN_POINT ( 'NONE',  ( 151.3258811035896656, 12.00000000000000000, -56.13263083939798292 ) ) ;
#1640=VERTEX_POINT ( 'NONE', #6105 ) ;
#1642=AXIS2_PLACEMENT_3D ( 'NONE', #6288, #7280, #1721 ) ;
#1644=CYLINDRICAL_SURFACE ( 'NONE', #11719, 134.9999999999999716 ) ;
#1650=AXIS2_PLACEMENT_3D ( 'NONE', #6841, #10610, #2149 ) ;
#1654=VERTEX_POINT ( 'NONE', #1583 ) ;
#1657=CYLINDRICAL_SURFACE ( 'NONE', #6275, 7.500000000000007105 ) ;
#1658=CARTESIAN_POINT ( 'NONE',  ( 35.00000000000000000, 81.99999999999998579, 190.3192290001959748 ) ) ;
#1662=ORIENTED_EDGE ( 'NONE', *, *, #4942, .F. ) ;
#1664=DIRECTION ( 'NONE',  ( -0.000000000000000000, -1.000000000000000000, -0.000000000000000000 ) ) ;
#1665=DIRECTION ( 'NONE',  ( 0.000000000000000000, 0.000000000000000000, 1.000000000000000000 ) ) ;
#1670=LINE ( 'NONE', #3569, #9944 ) ;
#1673=FACE_OUTER_BOUND ( 'NONE', #5768, .T. ) ;
#1674=ORIENTED_EDGE ( 'NONE', *, *, #10837, .F. ) ;
#1675=CARTESIAN_POINT ( 'NONE',  ( 1.561981751485805177E-12, -6.000000000000006217, 31.07864376269051121 ) ) ;
#1676=( LENGTH_UNIT ( ) NAMED_UNIT ( * ) SI_UNIT ( .MILLI., .METRE. ) );
#1678=DIRECTION ( 'NONE',  ( 0.000000000000000000, 0.000000000000000000, 1.000000000000000000 ) ) ;
#1683=AXIS2_PLACEMENT_3D ( 'NONE', #3512, #2593, #6365 ) ;
#1687=EDGE_LOOP ( 'NONE', ( #5931, #3580 ) ) ;
#1691=AXIS2_PLACEMENT_3D ( 'NONE', #11611, #2622, #6400 ) ;
#1694=DIRECTION ( 'NONE',  ( 0.000000000000000000, 0.000000000000000000, 1.000000000000000000 ) ) ;
#1702=VERTEX_POINT ( 'NONE', #9184 ) ;
#1706=CARTESIAN_POINT ( 'NONE',  ( 35.00000000000000000, 12.00000000000000000, 81.78351099501843180 ) ) ;
#1709=FACE_OUTER_BOUND ( 'NONE', #4848, .T. ) ;
#1713=CARTESIAN_POINT ( 'NONE',  ( 0.000000000000000000, 12.00000000000000000, -89.68077099980401101 ) ) ;
#1720=ORIENTED_EDGE ( 'NONE', *, *, #564, .T. ) ;
#1721=DIRECTION ( 'NONE',  ( 0.000000000000000000, 0.000000000000000000, 1.000000000000000000 ) ) ;
#1724=CARTESIAN_POINT ( 'NONE',  ( 35.00000000000000000, 164.0000000000000000, -124.6807709998038689 ) ) ;
#1725=AXIS2_PLACEMENT_3D ( 'NONE', #2506, #656, #3488 ) ;
#1738=DIRECTION ( 'NONE',  ( 0.000000000000000000, 0.000000000000000000, 1.000000000000000000 ) ) ;
#1743=FACE_OUTER_BOUND ( 'NONE', #3927, .T. ) ;
#1749=CARTESIAN_POINT ( 'NONE',  ( 1.250503886288004501E-12, -6.000000000000004441, -13.92135623730950478 ) ) ;
#1750=EDGE_LOOP ( 'NONE', ( #6442, #1267 ) ) ;
#1751=AXIS2_PLACEMENT_3D ( 'NONE', #7084, #2387, #3243 ) ;
#1752=AXIS2_PLACEMENT_3D ( 'NONE', #8038, #540, #7288 ) ;
#1754=CARTESIAN_POINT ( 'NONE',  ( 6.247927005943220505E-13, 12.00000000000000000, -66.42135623730949590 ) ) ;
#1757=DIRECTION ( 'NONE',  ( -0.000000000000000000, 1.000000000000000000, 0.000000000000000000 ) ) ;
#1759=VECTOR ( 'NONE', #7848, 1000.000000000000000 ) ;
#1764=CARTESIAN_POINT ( 'NONE',  ( 1.874378101782966050E-12, 12.00000000000000000, 61.07864376269051121 ) ) ;
#1766=CIRCLE ( 'NONE', #1563, 7.500000000000007105 ) ;
#1773=ORIENTED_EDGE ( 'NONE', *, *, #6240, .T. ) ;
#1777=AXIS2_PLACEMENT_3D ( 'NONE', #9816, #356, #6913 ) ;
#1779=DIRECTION ( 'NONE',  ( -0.000000000000000000, -7.930164461608263644E-17, 1.000000000000000000 ) ) ;
#1781=CYLINDRICAL_SURFACE ( 'NONE', #8687, 7.500000000000007994 ) ;
#1792=EDGE_CURVE ( 'NONE', #10730, #2533, #9136, .T. ) ;
#1793=ORIENTED_EDGE ( 'NONE', *, *, #6606, .F. ) ;
#1795=CYLINDRICAL_SURFACE ( 'NONE', #10448, 7.500000000000007105 ) ;
#1807=ORIENTED_EDGE ( 'NONE', *, *, #7454, .T. ) ;
#1812=ADVANCED_FACE ( 'NONE', ( #10178 ), #1644, .F. ) ;
#1825=DIRECTION ( 'NONE',  ( 0.000000000000000000, 0.000000000000000000, 1.000000000000000000 ) ) ;
#1838=LINE ( 'NONE', #5602, #8379 ) ;
#1843=DIRECTION ( 'NONE',  ( 0.000000000000000000, 0.000000000000000000, 1.000000000000000000 ) ) ;
#1844=EDGE_CURVE ( 'NONE', #1455, #7353, #10299, .T. ) ;
#1845=ORIENTED_EDGE ( 'NONE', *, *, #3755, .F. ) ;
#1846=DIRECTION ( 'NONE',  ( 0.000000000000000000, 1.000000000000000000, 0.000000000000000000 ) ) ;
#1847=EDGE_CURVE ( 'NONE', #7181, #4605, #1838, .T. ) ;
#1848=AXIS2_PLACEMENT_3D ( 'NONE', #4997, #2109, #4085 ) ;
#1856=VERTEX_POINT ( 'NONE', #9497 ) ;
#1861=DIRECTION ( 'NONE',  ( 0.000000000000000000, 1.000000000000000000, 0.000000000000000000 ) ) ;
#1863=VERTEX_POINT ( 'NONE', #10604 ) ;
#1864=FACE_OUTER_BOUND ( 'NONE', #7942, .T. ) ;
#1866=ADVANCED_FACE ( 'NONE', ( #974 ), #3805, .T. ) ;
#1873=ORIENTED_EDGE ( 'NONE', *, *, #3334, .F. ) ;
#1886=AXIS2_PLACEMENT_3D ( 'NONE', #3034, #893, #9591 ) ;
#1887=VECTOR ( 'NONE', #3375, 1000.000000000000000 ) ;
#1889=DIRECTION ( 'NONE',  ( 0.000000000000000000, 1.000000000000000000, 2.312964634635740689E-15 ) ) ;
#1895=FACE_BOUND ( 'NONE', #6123, .T. ) ;
#1903=ORIENTED_EDGE ( 'NONE', *, *, #2818, .T. ) ;
#1909=AXIS2_PLACEMENT_3D ( 'NONE', #1145, #4899, #3790 ) ;
#1915=AXIS2_PLACEMENT_3D ( 'NONE', #4118, #3178, #2808 ) ;
#1919=DIRECTION ( 'NONE',  ( 0.000000000000000000, 0.000000000000000000, 1.000000000000000000 ) ) ;
#1929=EDGE_CURVE ( 'NONE', #9223, #6290, #4213, .T. ) ;
#1930=EDGE_LOOP ( 'NONE', ( #1720, #11297, #5027, #837 ) ) ;
#1932=EDGE_CURVE ( 'NONE', #11819, #8540, #4406, .T. ) ;
#1936=VERTEX_POINT ( 'NONE', #12233 ) ;
#1943=EDGE_CURVE ( 'NONE', #338, #9776, #5982, .T. ) ;
#1944=DIRECTION ( 'NONE',  ( 0.000000000000000000, 0.000000000000000000, 1.000000000000000000 ) ) ;
#1955=VECTOR ( 'NONE', #11204, 1000.000000000000000 ) ;
#1964=DIRECTION ( 'NONE',  ( 0.000000000000000000, 1.000000000000000000, 0.000000000000000000 ) ) ;
#1965=AXIS2_PLACEMENT_3D ( 'NONE', #11493, #7661, #5795 ) ;
#1967=DIRECTION ( 'NONE',  ( 0.000000000000000000, 0.000000000000000000, -1.000000000000000000 ) ) ;
#1976=CARTESIAN_POINT ( 'NONE',  ( 0.000000000000000000, 12.00000000000000000, -89.68077099980401101 ) ) ;
#1980=ORIENTED_EDGE ( 'NONE', *, *, #1201, .F. ) ;
#1985=DIRECTION ( 'NONE',  ( 0.000000000000000000, 1.000000000000000000, 0.000000000000000000 ) ) ;
#1991=ORIENTED_EDGE ( 'NONE', *, *, #2465, .T. ) ;
#1992=ORIENTED_EDGE ( 'NONE', *, *, #8592, .T. ) ;
#1997=ORIENTED_EDGE ( 'NONE', *, *, #898, .F. ) ;
#1998=EDGE_CURVE ( 'NONE', #5359, #6447, #5782, .T. ) ;
#2002=ADVANCED_FACE ( 'NONE', ( #11048 ), #7528, .F. ) ;
#2003=CARTESIAN_POINT ( 'NONE',  ( 35.00000000000000000, 81.99999999999998579, 190.3192290001959748 ) ) ;
#2007=CARTESIAN_POINT ( 'NONE',  ( 1.562900236585165577E-12, 12.00000000000000000, 16.07864376269049700 ) ) ;
#2010=EDGE_LOOP ( 'NONE', ( #6975, #4556 ) ) ;
#2018=EDGE_CURVE ( 'NONE', #3679, #10836, #2419, .T. ) ;
#2033=CARTESIAN_POINT ( 'NONE',  ( 3.133148353965215262E-13, -6.000000000000004441, -103.9213562373094959 ) ) ;
#2035=DIRECTION ( 'NONE',  ( 0.000000000000000000, 1.000000000000000000, 0.000000000000000000 ) ) ;
#2040=CARTESIAN_POINT ( 'NONE',  ( 35.00000000000000000, 163.9999999999999716, 190.3192290001959748 ) ) ;
#2041=LINE ( 'NONE', #11434, #11152 ) ;
#2043=LINE ( 'NONE', #8874, #9637 ) ;
#2054=CIRCLE ( 'NONE', #12131, 7.500000000000013323 ) ;
#2055=VERTEX_POINT ( 'NONE', #10429 ) ;
#2056=CIRCLE ( 'NONE', #8389, 7.500000000000007105 ) ;
#2063=CIRCLE ( 'NONE', #672, 7.500000000000007105 ) ;
#2076=VERTEX_POINT ( 'NONE', #2094 ) ;
#2077=CARTESIAN_POINT ( 'NONE',  ( 1.479627290717497352E-14, 152.0000000000000284, 118.9213562373094817 ) ) ;
#2082=CIRCLE ( 'NONE', #3440, 7.500000000000013323 ) ;
#2092=ADVANCED_FACE ( 'NONE', ( #4806 ), #8702, .F. ) ;
#2093=VERTEX_POINT ( 'NONE', #1221 ) ;
#2094=CARTESIAN_POINT ( 'NONE',  ( 3.123963502971610252E-13, 12.00000000000000000, -88.92135623730948168 ) ) ;
#2101=CARTESIAN_POINT ( 'NONE',  ( 1.875296586882326249E-12, 152.0000000000000000, 46.07864376269051121 ) ) ;
#2109=DIRECTION ( 'NONE',  ( 0.000000000000000000, -1.000000000000000000, -7.930164461608263644E-17 ) ) ;
#2111=FACE_BOUND ( 'NONE', #9135, .T. ) ;
#2113=VECTOR ( 'NONE', #908, 1000.000000000000000 ) ;
#2116=DIRECTION ( 'NONE',  ( 0.000000000000000000, 0.000000000000000000, 1.000000000000000000 ) ) ;
#2124=DIRECTION ( 'NONE',  ( 0.000000000000000000, 0.000000000000000000, -1.000000000000000000 ) ) ;
#2127=CIRCLE ( 'NONE', #8642, 7.500000000000007105 ) ;
#2128=CARTESIAN_POINT ( 'NONE',  ( 6.247927005943220505E-13, -6.000000000000006217, -58.92135623730948879 ) ) ;
#2137=EDGE_LOOP ( 'NONE', ( #5105, #4327, #5467, #4968 ) ) ;
#2149=DIRECTION ( 'NONE',  ( 0.000000000000000000, 0.000000000000000000, -1.000000000000000000 ) ) ;
#2158=DIRECTION ( 'NONE',  ( -1.000000000000000000, -0.000000000000000000, 0.000000000000000000 ) ) ;
#2161=DIRECTION ( 'NONE',  ( 0.000000000000000000, 0.000000000000000000, 1.000000000000000000 ) ) ;
#2170=VERTEX_POINT ( 'NONE', #11608 ) ;
#2172=EDGE_CURVE ( 'NONE', #10880, #11915, #3222, .T. ) ;
#2174=LINE ( 'NONE', #5937, #7546 ) ;
#2175=ORIENTED_EDGE ( 'NONE', *, *, #11470, .F. ) ;
#2176=ORIENTED_EDGE ( 'NONE', *, *, #8867, .T. ) ;
#2184=CARTESIAN_POINT ( 'NONE',  ( -151.3258811035894098, 12.00000000000000000, -56.13263083939680342 ) ) ;
#2187=ORIENTED_EDGE ( 'NONE', *, *, #4356, .F. ) ;
#2194=VERTEX_POINT ( 'NONE', #10728 ) ;
#2199=DIRECTION ( 'NONE',  ( 0.000000000000000000, 0.000000000000000000, 1.000000000000000000 ) ) ;
#2203=ORIENTED_EDGE ( 'NONE', *, *, #11459, .T. ) ;
#2205=ORIENTED_EDGE ( 'NONE', *, *, #944, .T. ) ;
#2207=ORIENTED_EDGE ( 'NONE', *, *, #9846, .F. ) ;
#2210=CARTESIAN_POINT ( 'NONE',  ( 1.875296586882326249E-12, -6.000000000000004441, 46.07864376269049700 ) ) ;
#2212=CIRCLE ( 'NONE', #11498, 7.500000000000013323 ) ;
#2213=ADVANCED_FACE ( 'NONE', ( #8984 ), #1394, .F. ) ;
#2219=DIRECTION ( 'NONE',  ( 0.000000000000000000, 1.000000000000000000, 0.000000000000000000 ) ) ;
#2223=ADVANCED_FACE ( 'NONE', ( #7138 ), #5158, .F. ) ;
#2224=DIRECTION ( 'NONE',  ( -0.000000000000000000, 1.000000000000000000, 7.930164461608263644E-17 ) ) ;
#2226=DIRECTION ( 'NONE',  ( 0.000000000000000000, 1.000000000000000000, 0.000000000000000000 ) ) ;
#2229=ORIENTED_EDGE ( 'NONE', *, *, #8271, .F. ) ;
#2235=ADVANCED_FACE ( 'NONE', ( #5972 ), #1285, .F. ) ;
#2243=VECTOR ( 'NONE', #1586, 1000.000000000000000 ) ;
#2250=CARTESIAN_POINT ( 'NONE',  ( 1.561981751485805177E-12, 12.00000000000000000, 23.57864376269050410 ) ) ;
#2253=CARTESIAN_POINT ( 'NONE',  ( -6.106226635438360972E-13, 12.00000000000000000, -244.6807709998039400 ) ) ;
#2274=FACE_OUTER_BOUND ( 'NONE', #11529, .T. ) ;
#2275=AXIS2_PLACEMENT_3D ( 'NONE', #3443, #10192, #3500 ) ;
#2277=CARTESIAN_POINT ( 'NONE',  ( -45.53315400109751465, 0.000000000000000000, -237.8419396193594650 ) ) ;
#2278=FACE_BOUND ( 'NONE', #8897, .T. ) ;
#2282=VERTEX_POINT ( 'NONE', #8256 ) ;
#2286=EDGE_CURVE ( 'NONE', #694, #3418, #4234, .T. ) ;
#2290=FACE_BOUND ( 'NONE', #6621, .T. ) ;
#2297=DIRECTION ( 'NONE',  ( -0.000000000000000000, 1.000000000000000000, 7.930164461608263644E-17 ) ) ;
#2298=ORIENTED_EDGE ( 'NONE', *, *, #8213, .T. ) ;
#2299=EDGE_CURVE ( 'NONE', #5668, #7181, #7507, .T. ) ;
#2306=ADVANCED_FACE ( 'NONE', ( #11334 ), #6639, .F. ) ;
#2314=ORIENTED_EDGE ( 'NONE', *, *, #7359, .F. ) ;
#2326=ORIENTED_EDGE ( 'NONE', *, *, #11602, .T. ) ;
#2337=AXIS2_PLACEMENT_3D ( 'NONE', #8289, #2518, #5294 ) ;
#2340=CARTESIAN_POINT ( 'NONE',  ( -154.5043356068770493, 12.00000000000000000, -94.56666130601601594 ) ) ;
#2341=CARTESIAN_POINT ( 'NONE',  ( 126.4213562373094959, 0.000000000000000000, 7.500000000000007105 ) ) ;
#2347=EDGE_LOOP ( 'NONE', ( #8247, #110 ) ) ;
#2351=FACE_OUTER_BOUND ( 'NONE', #3276, .T. ) ;
#2353=ORIENTED_EDGE ( 'NONE', *, *, #2018, .T. ) ;
#2354=AXIS2_PLACEMENT_3D ( 'NONE', #8145, #6171, #3369 ) ;
#2360=DIRECTION ( 'NONE',  ( 1.000000000000000000, 0.000000000000000000, -0.000000000000000000 ) ) ;
#2362=FILL_AREA_STYLE ('',( #2597 ) ) ;
#2366=ORIENTED_EDGE ( 'NONE', *, *, #7290, .F. ) ;
#2370=EDGE_CURVE ( 'NONE', #10860, #918, #6195, .T. ) ;
#2372=EDGE_LOOP ( 'NONE', ( #7598, #10524, #2572, #9505, #11703 ) ) ;
#2378=VERTEX_POINT ( 'NONE', #1764 ) ;
#2383=DIRECTION ( 'NONE',  ( 0.000000000000000000, 0.000000000000000000, 1.000000000000000000 ) ) ;
#2384=EDGE_LOOP ( 'NONE', ( #173, #10384, #8616, #4301 ) ) ;
#2387=DIRECTION ( 'NONE',  ( -0.000000000000000000, -1.000000000000000000, -0.000000000000000000 ) ) ;
#2389=DIRECTION ( 'NONE',  ( 0.000000000000000000, -1.156482317317870246E-16, 1.000000000000000000 ) ) ;
#2416=ORIENTED_EDGE ( 'NONE', *, *, #8925, .T. ) ;
#2419=CIRCLE ( 'NONE', #10913, 7.500000000000007105 ) ;
#2422=ORIENTED_EDGE ( 'NONE', *, *, #4862, .F. ) ;
#2427=EDGE_CURVE ( 'NONE', #9404, #1455, #6387, .T. ) ;
#2429=LINE ( 'NONE', #6209, #11195 ) ;
#2436=EDGE_LOOP ( 'NONE', ( #386, #34 ) ) ;
#2437=CARTESIAN_POINT ( 'NONE',  ( 2.186774452080127126E-12, -6.000000000000005329, 83.57864376269050410 ) ) ;
#2440=ORIENTED_EDGE ( 'NONE', *, *, #2696, .T. ) ;
#2441=DIRECTION ( 'NONE',  ( 0.000000000000000000, -1.000000000000000000, -7.930164461608263644E-17 ) ) ;
#2447=EDGE_CURVE ( 'NONE', #10609, #8307, #5789, .T. ) ;
#2451=CARTESIAN_POINT ( 'NONE',  ( -35.00000000000000000, -4.436643353671145300E-15, 81.78351099501843180 ) ) ;
#2453=PLANE ( 'NONE',  #1333 ) ;
#2456=LINE ( 'NONE', #2638, #5868 ) ;
#2458=AXIS2_PLACEMENT_3D ( 'NONE', #1153, #5835, #9787 ) ;
#2459=CIRCLE ( 'NONE', #5417, 7.500000000000007105 ) ;
#2464=ORIENTED_EDGE ( 'NONE', *, *, #10327, .T. ) ;
#2465=EDGE_CURVE ( 'NONE', #5569, #6750, #1257, .T. ) ;
#2468=CIRCLE ( 'NONE', #4264, 7.500000000000013323 ) ;
#2470=PLANE ( 'NONE',  #11143 ) ;
#2475=FACE_OUTER_BOUND ( 'NONE', #11339, .T. ) ;
#2477=VERTEX_POINT ( 'NONE', #992 ) ;
#2481=ORIENTED_EDGE ( 'NONE', *, *, #3995, .F. ) ;
#2488=CIRCLE ( 'NONE', #6244, 7.500000000000013323 ) ;
#2491=DIRECTION ( 'NONE',  ( 0.000000000000000000, 0.000000000000000000, 1.000000000000000000 ) ) ;
#2492=AXIS2_PLACEMENT_3D ( 'NONE', #3606, #9245, #26 ) ;
#2496=EDGE_CURVE ( 'NONE', #8307, #10609, #9740, .T. ) ;
#2498=ORIENTED_EDGE ( 'NONE', *, *, #2855, .F. ) ;
#2504=CIRCLE ( 'NONE', #2917, 7.500000000000007105 ) ;
#2506=CARTESIAN_POINT ( 'NONE',  ( -126.4213562373094959, 12.00000000000000000, 2.255140518769849223E-14 ) ) ;
#2508=CARTESIAN_POINT ( 'NONE',  ( 87.04832655144112152, 0.000000000000000000, -225.4289243767383368 ) ) ;
#2509=DIRECTION ( 'NONE',  ( 0.000000000000000000, 1.000000000000000000, 0.000000000000000000 ) ) ;
#2511=FACE_BOUND ( 'NONE', #8042, .T. ) ;
#2512=CARTESIAN_POINT ( 'NONE',  ( 2.186774452080127126E-12, -6.000000000000005329, 83.57864376269050410 ) ) ;
#2514=VERTEX_POINT ( 'NONE', #4988 ) ;
#2517=CYLINDRICAL_SURFACE ( 'NONE', #10894, 7.500000000000007105 ) ;
#2518=DIRECTION ( 'NONE',  ( -0.000000000000000000, -1.000000000000000000, -0.000000000000000000 ) ) ;
#2533=VERTEX_POINT ( 'NONE', #2101 ) ;
#2537=CARTESIAN_POINT ( 'NONE',  ( 3.123963502971610252E-13, 152.0000000000000000, -88.92135623730946747 ) ) ;
#2539=VECTOR ( 'NONE', #5120, 1000.000000000000000 ) ;
#2542=ADVANCED_FACE ( 'NONE', ( #4931 ), #226, .F. ) ;
#2543=EDGE_CURVE ( 'NONE', #6290, #9223, #2054, .T. ) ;
#2550=EDGE_LOOP ( 'NONE', ( #8471, #8703, #7056, #11086 ) ) ;
#2553=ORIENTED_EDGE ( 'NONE', *, *, #11769, .F. ) ;
#2555=AXIS2_PLACEMENT_3D ( 'NONE', #8142, #7215, #10983 ) ;
#2556=CARTESIAN_POINT ( 'NONE',  ( -151.3258811035894098, 12.00000000000000000, -56.13263083939680342 ) ) ;
#2561=FACE_OUTER_BOUND ( 'NONE', #4749, .T. ) ;
#2567=DIRECTION ( 'NONE',  ( -0.000000000000000000, 1.000000000000000000, 0.000000000000000000 ) ) ;
#2569=CARTESIAN_POINT ( 'NONE',  ( 1.387778780781445676E-14, 152.0000000000000284, 126.4213562373094959 ) ) ;
#2572=ORIENTED_EDGE ( 'NONE', *, *, #8792, .T. ) ;
#2573=DIRECTION ( 'NONE',  ( 0.000000000000000000, 0.000000000000000000, -1.000000000000000000 ) ) ;
#2578=CIRCLE ( 'NONE', #7719, 7.500000000000007105 ) ;
#2579=DIRECTION ( 'NONE',  ( -0.000000000000000000, 1.000000000000000000, -0.000000000000000000 ) ) ;
#2581=EDGE_CURVE ( 'NONE', #6447, #5359, #2063, .T. ) ;
#2583=EDGE_CURVE ( 'NONE', #11133, #2514, #6986, .T. ) ;
#2592=DIRECTION ( 'NONE',  ( 0.000000000000000000, 0.000000000000000000, 1.000000000000000000 ) ) ;
#2593=DIRECTION ( 'NONE',  ( -0.000000000000000000, 1.000000000000000000, 7.930164461608263644E-17 ) ) ;
#2597=FILL_AREA_STYLE_COLOUR ( '', #8264 ) ;
#2603=VERTEX_POINT ( 'NONE', #11854 ) ;
#2606=ORIENTED_EDGE ( 'NONE', *, *, #4478, .F. ) ;
#2609=EDGE_LOOP ( 'NONE', ( #3465, #10628, #4567, #1129 ) ) ;
#2612=DIRECTION ( 'NONE',  ( -0.000000000000000000, 1.000000000000000000, 7.930164461608263644E-17 ) ) ;
#2615=EDGE_CURVE ( 'NONE', #6173, #4980, #11332, .T. ) ;
#2617=CARTESIAN_POINT ( 'NONE',  ( -120.8820948793972434, 0.000000000000000000, -179.1989091883324363 ) ) ;
#2620=VERTEX_POINT ( 'NONE', #660 ) ;
#2622=DIRECTION ( 'NONE',  ( 0.000000000000000000, 1.000000000000000000, 0.000000000000000000 ) ) ;
#2623=ORIENTED_EDGE ( 'NONE', *, *, #2286, .T. ) ;
#2624=CARTESIAN_POINT ( 'NONE',  ( 151.3258811035896656, 12.00000000000000000, -63.63263083939799003 ) ) ;
#2628=DIRECTION ( 'NONE',  ( 0.000000000000000000, 0.000000000000000000, 1.000000000000000000 ) ) ;
#2633=AXIS2_PLACEMENT_3D ( 'NONE', #1340, #5039, #4175 ) ;
#2634=ORIENTED_EDGE ( 'NONE', *, *, #1943, .F. ) ;
#2637=ORIENTED_EDGE ( 'NONE', *, *, #5912, .F. ) ;
#2638=CARTESIAN_POINT ( 'NONE',  ( 45.53315400109643463, 12.00000000000000000, -230.3419396193597208 ) ) ;
#2641=CARTESIAN_POINT ( 'NONE',  ( 1.561981751485805177E-12, 152.0000000000000000, 31.07864376269052542 ) ) ;
#2644=VECTOR ( 'NONE', #6740, 1000.000000000000000 ) ;
#2649=ORIENTED_EDGE ( 'NONE', *, *, #7463, .F. ) ;
#2654=EDGE_CURVE ( 'NONE', #4090, #11527, #10941, .T. ) ;
#2660=CARTESIAN_POINT ( 'NONE',  ( 1.874378101782966050E-12, 0.000000000000000000, 53.57864376269050410 ) ) ;
#2661=ORIENTED_EDGE ( 'NONE', *, *, #9929, .T. ) ;
#2678=ORIENTED_EDGE ( 'NONE', *, *, #10006, .F. ) ;
#2679=DIRECTION ( 'NONE',  ( 0.000000000000000000, 0.000000000000000000, 1.000000000000000000 ) ) ;
#2680=EDGE_CURVE ( 'NONE', #10476, #2514, #9189, .T. ) ;
#2683=VECTOR ( 'NONE', #11928, 1000.000000000000000 ) ;
#2685=CARTESIAN_POINT ( 'NONE',  ( 0.000000000000000000, 12.00000000000000000, -224.6807709998039968 ) ) ;
#2691=DIRECTION ( 'NONE',  ( 0.000000000000000000, 1.000000000000000000, 0.000000000000000000 ) ) ;
#2694=DIRECTION ( 'NONE',  ( 0.000000000000000000, 1.000000000000000000, 0.000000000000000000 ) ) ;
#2696=EDGE_CURVE ( 'NONE', #6669, #1396, #3834, .T. ) ;
#2706=DIRECTION ( 'NONE',  ( -0.000000000000000000, 1.000000000000000000, 7.930164461608263644E-17 ) ) ;
#2708=ORIENTED_EDGE ( 'NONE', *, *, #5618, .T. ) ;
#2710=EDGE_CURVE ( 'NONE', #5191, #6316, #6595, .T. ) ;
#2712=CARTESIAN_POINT ( 'NONE',  ( 2.186774452080127126E-12, -6.000000000000006217, 91.07864376269050410 ) ) ;
#2715=ORIENTED_EDGE ( 'NONE', *, *, #6765, .T. ) ;
#2720=FACE_OUTER_BOUND ( 'NONE', #9967, .T. ) ;
#2726=EDGE_LOOP ( 'NONE', ( #3973, #10532 ) ) ;
#2733=VERTEX_POINT ( 'NONE', #9062 ) ;
#2736=AXIS2_PLACEMENT_3D ( 'NONE', #6664, #7654, #3697 ) ;
#2738=CARTESIAN_POINT ( 'NONE',  ( -35.00000000000000000, 81.99999999999998579, 190.3192290001959748 ) ) ;
#2742=CARTESIAN_POINT ( 'NONE',  ( 126.4213562373094959, 12.00000000000000000, -6.938893903907228378E-15 ) ) ;
#2743=FACE_OUTER_BOUND ( 'NONE', #9647, .T. ) ;
#2744=ORIENTED_EDGE ( 'NONE', *, *, #10471, .T. ) ;
#2746=DIRECTION ( 'NONE',  ( -0.000000000000000000, 1.000000000000000000, 0.000000000000000000 ) ) ;
#2751=CIRCLE ( 'NONE', #5707, 7.500000000000020428 ) ;
#2760=EDGE_CURVE ( 'NONE', #8440, #6717, #10736, .T. ) ;
#2765=VECTOR ( 'NONE', #6050, 1000.000000000000000 ) ;
#2766=AXIS2_PLACEMENT_3D ( 'NONE', #2569, #11972, #722 ) ;
#2776=EDGE_LOOP ( 'NONE', ( #9375, #9900, #37, #10500 ) ) ;
#2784=DIRECTION ( 'NONE',  ( 0.000000000000000000, 0.000000000000000000, 1.000000000000000000 ) ) ;
#2787=CARTESIAN_POINT ( 'NONE',  ( 9.184850993605159777E-16, -58.00000000000000711, -133.9213562373095101 ) ) ;
#2788=SHAPE_REPRESENTATION_RELATIONSHIP ( 'NONE' , 'NONE' ,  #4488, #3228 ) ;
#2793=EDGE_LOOP ( 'NONE', ( #1256, #116 ) ) ;
#2797=ORIENTED_EDGE ( 'NONE', *, *, #5643, .F. ) ;
#2798=CIRCLE ( 'NONE', #10491, 7.500000000000007105 ) ;
#2808=DIRECTION ( 'NONE',  ( 0.000000000000000000, 0.000000000000000000, 1.000000000000000000 ) ) ;
#2812=CARTESIAN_POINT ( 'NONE',  ( 45.53315400109643463, 12.00000000000000000, -245.3419396193597493 ) ) ;
#2813=DIRECTION ( 'NONE',  ( 0.000000000000000000, 0.000000000000000000, 1.000000000000000000 ) ) ;
#2817=DIRECTION ( 'NONE',  ( 0.000000000000000000, 7.930164461608263644E-17, -1.000000000000000000 ) ) ;
#2818=EDGE_CURVE ( 'NONE', #3744, #10023, #4640, .T. ) ;
#2824=CARTESIAN_POINT ( 'NONE',  ( 1.874378101782966050E-12, 152.0000000000000000, 53.57864376269051832 ) ) ;
#2833=VECTOR ( 'NONE', #9248, 1000.000000000000000 ) ;
#2838=CARTESIAN_POINT ( 'NONE',  ( -35.00000000000000000, 152.0000000000000000, 190.3192290001959748 ) ) ;
#2839=CARTESIAN_POINT ( 'NONE',  ( -6.097041784444755962E-13, 0.000000000000000000, -237.1807709998039115 ) ) ;
#2840=EDGE_CURVE ( 'NONE', #1396, #6669, #3045, .T. ) ;
#2842=AXIS2_PLACEMENT_3D ( 'NONE', #3082, #2035, #2161 ) ;
#2844=ORIENTED_EDGE ( 'NONE', *, *, #9479, .F. ) ;
#2845=DIRECTION ( 'NONE',  ( 0.000000000000000000, 1.000000000000000000, 0.000000000000000000 ) ) ;
#2855=EDGE_CURVE ( 'NONE', #5146, #9369, #11014, .T. ) ;
#2857=EDGE_CURVE ( 'NONE', #4489, #2055, #7391, .T. ) ;
#2862=CARTESIAN_POINT ( 'NONE',  ( -35.00000000000000000, 12.00000000000000000, 81.78351099501843180 ) ) ;
#2864=VECTOR ( 'NONE', #11991, 1000.000000000000000 ) ;
#2865=AXIS2_PLACEMENT_3D ( 'NONE', #8919, #10847, #9921 ) ;
#2873=DIRECTION ( 'NONE',  ( -0.000000000000000000, 1.000000000000000000, 7.930164461608263644E-17 ) ) ;
#2874=AXIS2_PLACEMENT_3D ( 'NONE', #5585, #2746, #907 ) ;
#2875=CARTESIAN_POINT ( 'NONE',  ( 0.000000000000000000, 12.00000000000001954, -124.6807709998040110 ) ) ;
#2891=DIRECTION ( 'NONE',  ( 0.000000000000000000, -2.379049338482476554E-15, 1.000000000000000000 ) ) ;
#2893=EDGE_CURVE ( 'NONE', #8366, #10273, #9747, .T. ) ;
#2900=DIRECTION ( 'NONE',  ( -1.000000000000000000, -0.000000000000000000, 0.000000000000000000 ) ) ;
#2907=EDGE_CURVE ( 'NONE', #1863, #83, #7787, .T. ) ;
#2908=AXIS2_PLACEMENT_3D ( 'NONE', #6518, #8191, #11278 ) ;
#2913=DIRECTION ( 'NONE',  ( 0.000000000000000000, 0.000000000000000000, 1.000000000000000000 ) ) ;
#2917=AXIS2_PLACEMENT_3D ( 'NONE', #8192, #5455, #9171 ) ;
#2918=FACE_BOUND ( 'NONE', #890, .T. ) ;
#2921=VERTEX_POINT ( 'NONE', #10334 ) ;
#2922=CARTESIAN_POINT ( 'NONE',  ( 1.387778780781445676E-14, 163.9999999999999716, 133.9213562373095101 ) ) ;
#2929=CARTESIAN_POINT ( 'NONE',  ( 1.874378101782966050E-12, -6.000000000000005329, 53.57864376269050410 ) ) ;
#2935=FACE_OUTER_BOUND ( 'NONE', #1143, .T. ) ;
#2940=VECTOR ( 'NONE', #9312, 1000.000000000000000 ) ;
#2943=CIRCLE ( 'NONE', #3928, 7.500000000000007105 ) ;
#2945=ORIENTED_EDGE ( 'NONE', *, *, #9759, .F. ) ;
#2954=ORIENTED_EDGE ( 'NONE', *, *, #6853, .T. ) ;
#2956=ORIENTED_EDGE ( 'NONE', *, *, #8524, .F. ) ;
#2959=CARTESIAN_POINT ( 'NONE',  ( -45.53315400109751465, 12.00000000000000000, -230.3419396193594366 ) ) ;
#2964=DIRECTION ( 'NONE',  ( 0.000000000000000000, 0.000000000000000000, 1.000000000000000000 ) ) ;
#2968=FACE_OUTER_BOUND ( 'NONE', #3173, .T. ) ;
#2969=ORIENTED_EDGE ( 'NONE', *, *, #1929, .F. ) ;
#2976=EDGE_CURVE ( 'NONE', #502, #5191, #1135, .T. ) ;
#2981=ORIENTED_EDGE ( 'NONE', *, *, #9759, .T. ) ;
#2983=DIRECTION ( 'NONE',  ( -0.000000000000000000, 1.000000000000000000, 7.930164461608263644E-17 ) ) ;
#2985=DIRECTION ( 'NONE',  ( 0.000000000000000000, 0.000000000000000000, 1.000000000000000000 ) ) ;
#2986=CARTESIAN_POINT ( 'NONE',  ( 1.874378101782966050E-12, 163.9999999999999716, 53.57864376269051832 ) ) ;
#2989=AXIS2_PLACEMENT_3D ( 'NONE', #3408, #10165, #645 ) ;
#2992=CARTESIAN_POINT ( 'NONE',  ( -45.53315400109751465, 12.00000000000000000, -245.3419396193594650 ) ) ;
#2999=CARTESIAN_POINT ( 'NONE',  ( 1.561981751485805177E-12, 0.000000000000000000, 31.07864376269051121 ) ) ;
#3000=LINE ( 'NONE', #8564, #8478 ) ;
#3003=ORIENTED_EDGE ( 'NONE', *, *, #9097, .F. ) ;
#3009=ADVANCED_FACE ( 'NONE', ( #2290, #6124, #11756, #484, #3451, #6183, #9077, #9013, #613, #9949 ), #2470, .F. ) ;
#3014=ORIENTED_EDGE ( 'NONE', *, *, #11620, .T. ) ;
#3024=DIRECTION ( 'NONE',  ( -0.000000000000000000, -1.000000000000000000, -0.000000000000000000 ) ) ;
#3025=CARTESIAN_POINT ( 'NONE',  ( 154.5043356068769071, 12.00000000000000000, -102.0666613060171386 ) ) ;
#3029=CIRCLE ( 'NONE', #9931, 7.500000000000007105 ) ;
#3030=CARTESIAN_POINT ( 'NONE',  ( 0.000000000000000000, 164.0000000000000000, -118.9213562373094817 ) ) ;
#3033=EDGE_CURVE ( 'NONE', #2921, #4476, #10815, .T. ) ;
#3034=CARTESIAN_POINT ( 'NONE',  ( 0.000000000000000000, 0.000000000000000000, -89.68077099980401101 ) ) ;
#3036=CARTESIAN_POINT ( 'NONE',  ( 35.00000000000000000, 81.99999999999998579, 190.3192290001959748 ) ) ;
#3038=ORIENTED_EDGE ( 'NONE', *, *, #11746, .T. ) ;
#3045=CIRCLE ( 'NONE', #74, 7.500000000000007105 ) ;
#3047=VECTOR ( 'NONE', #1183, 1000.000000000000000 ) ;
#3048=CIRCLE ( 'NONE', #463, 7.500000000000007105 ) ;
#3049=DIRECTION ( 'NONE',  ( -0.000000000000000000, 1.000000000000000000, -0.000000000000000000 ) ) ;
#3053=EDGE_CURVE ( 'NONE', #7042, #5557, #8955, .T. ) ;
#3054=VERTEX_POINT ( 'NONE', #3380 ) ;
#3069=DIRECTION ( 'NONE',  ( 0.000000000000000000, 1.000000000000000000, 0.000000000000000000 ) ) ;
#3082=CARTESIAN_POINT ( 'NONE',  ( 120.8820948793965186, 12.00000000000000000, -186.6989091883332890 ) ) ;
#3088=CARTESIAN_POINT ( 'NONE',  ( -144.0488662551579182, 12.00000000000000000, -154.4077238332691877 ) ) ;
#3096=FACE_OUTER_BOUND ( 'NONE', #3647, .T. ) ;
#3099=ORIENTED_EDGE ( 'NONE', *, *, #2680, .T. ) ;
#3102=CARTESIAN_POINT ( 'NONE',  ( 9.371890508914830252E-13, 12.00000000000000000, -36.42135623730949590 ) ) ;
#3103=CARTESIAN_POINT ( 'NONE',  ( 2.186774452080127126E-12, 163.9999999999999716, 91.07864376269051832 ) ) ;
#3105=ORIENTED_EDGE ( 'NONE', *, *, #1312, .T. ) ;
#3118=EDGE_CURVE ( 'NONE', #4288, #7504, #6490, .T. ) ;
#3119=CARTESIAN_POINT ( 'NONE',  ( -35.00000000000000000, 81.99999999999998579, 272.3192290001959464 ) ) ;
#3121=EDGE_CURVE ( 'NONE', #5146, #9670, #5013, .T. ) ;
#3134=CARTESIAN_POINT ( 'NONE',  ( 45.53315400109643463, 12.00000000000000000, -237.8419396193597208 ) ) ;
#3138=EDGE_LOOP ( 'NONE', ( #4798, #4827, #11360, #2969 ) ) ;
#3141=DIRECTION ( 'NONE',  ( -0.000000000000000000, -1.000000000000000000, -0.000000000000000000 ) ) ;
#3149=DIRECTION ( 'NONE',  ( -0.000000000000000000, 1.000000000000000000, 7.930164461608263644E-17 ) ) ;
#3153=DIRECTION ( 'NONE',  ( 0.000000000000000000, 0.000000000000000000, 1.000000000000000000 ) ) ;
#3154=ORIENTED_EDGE ( 'NONE', *, *, #8749, .T. ) ;
#3163=VERTEX_POINT ( 'NONE', #812 ) ;
#3169=EDGE_LOOP ( 'NONE', ( #8629, #5837, #5953, #4964 ) ) ;
#3172=DIRECTION ( 'NONE',  ( 0.000000000000000000, 1.000000000000000000, 0.000000000000000000 ) ) ;
#3173=EDGE_LOOP ( 'NONE', ( #6073, #498, #10667, #6357 ) ) ;
#3178=DIRECTION ( 'NONE',  ( 0.000000000000000000, 1.000000000000000000, 0.000000000000000000 ) ) ;
#3181=EDGE_CURVE ( 'NONE', #5780, #11075, #10198, .T. ) ;
#3182=ORIENTED_EDGE ( 'NONE', *, *, #8229, .F. ) ;
#3183=ADVANCED_FACE ( 'NONE', ( #2720 ), #8298, .F. ) ;
#3184=ORIENTED_EDGE ( 'NONE', *, *, #321, .T. ) ;
#3189=CARTESIAN_POINT ( 'NONE',  ( 3.133148353965215262E-13, 0.000000000000000000, -103.9213562373094959 ) ) ;
#3190=DIRECTION ( 'NONE',  ( -0.000000000000000000, -1.000000000000000000, -0.000000000000000000 ) ) ;
#3191=AXIS2_PLACEMENT_3D ( 'NONE', #8656, #1179, #5048 ) ;
#3192=AXIS2_PLACEMENT_3D ( 'NONE', #239, #4025, #11568 ) ;
#3204=DIRECTION ( 'NONE',  ( 0.000000000000000000, 1.000000000000000000, 0.000000000000000000 ) ) ;
#3206=DIRECTION ( 'NONE',  ( 0.000000000000000000, 0.000000000000000000, 1.000000000000000000 ) ) ;
#3217=DIRECTION ( 'NONE',  ( 0.000000000000000000, 0.000000000000000000, 1.000000000000000000 ) ) ;
#3218=ORIENTED_EDGE ( 'NONE', *, *, #5033, .T. ) ;
#3220=ORIENTED_EDGE ( 'NONE', *, *, #1457, .T. ) ;
#3221=DIRECTION ( 'NONE',  ( 0.000000000000000000, 0.000000000000000000, 1.000000000000000000 ) ) ;
#3222=CIRCLE ( 'NONE', #8943, 7.500000000000013323 ) ;
#3226=DIRECTION ( 'NONE',  ( 0.000000000000000000, 0.000000000000000000, -1.000000000000000000 ) ) ;
#3227=ORIENTED_EDGE ( 'NONE', *, *, #7371, .F. ) ;
#3228=ADVANCED_BREP_SHAPE_REPRESENTATION ( '', ( #8194, #11957 ), #6826 ) ;
#3239=ORIENTED_EDGE ( 'NONE', *, *, #3405, .F. ) ;
#3240=VECTOR ( 'NONE', #7946, 1000.000000000000000 ) ;
#3243=DIRECTION ( 'NONE',  ( 0.000000000000000000, 0.000000000000000000, -1.000000000000000000 ) ) ;
#3249=LINE ( 'NONE', #350, #9319 ) ;
#3253=FACE_BOUND ( 'NONE', #4939, .T. ) ;
#3258=DIRECTION ( 'NONE',  ( 0.000000000000000000, 0.000000000000000000, -1.000000000000000000 ) ) ;
#3260=DIRECTION ( 'NONE',  ( -0.000000000000000000, -1.000000000000000000, -0.000000000000000000 ) ) ;
#3261=DIRECTION ( 'NONE',  ( -0.000000000000000000, 1.000000000000000000, -0.000000000000000000 ) ) ;
#3264=EDGE_CURVE ( 'NONE', #10273, #8366, #11823, .T. ) ;
#3265=ORIENTED_EDGE ( 'NONE', *, *, #1613, .F. ) ;
#3267=CARTESIAN_POINT ( 'NONE',  ( 35.00000000000000000, 152.0000000000000000, 190.3192290001959748 ) ) ;
#3268=CYLINDRICAL_SURFACE ( 'NONE', #7817, 7.500000000000007105 ) ;
#3275=CYLINDRICAL_SURFACE ( 'NONE', #1360, 7.500000000000007105 ) ;
#3276=EDGE_LOOP ( 'NONE', ( #1213, #1176, #9743, #11116 ) ) ;
#3278=CIRCLE ( 'NONE', #10196, 7.500000000000007105 ) ;
#3285=CIRCLE ( 'NONE', #10398, 7.500000000000007105 ) ;
#3293=VECTOR ( 'NONE', #8127, 1000.000000000000000 ) ;
#3295=EDGE_CURVE ( 'NONE', #5214, #2170, #3315, .T. ) ;
#3299=DIRECTION ( 'NONE',  ( -0.000000000000000000, 1.000000000000000000, 7.930164461608263644E-17 ) ) ;
#3304=CYLINDRICAL_SURFACE ( 'NONE', #3653, 7.500000000000007105 ) ;
#3305=ORIENTED_EDGE ( 'NONE', *, *, #1613, .T. ) ;
#3309=CARTESIAN_POINT ( 'NONE',  ( -35.00000000000000000, 81.99999999999998579, 190.3192290001959748 ) ) ;
#3311=DIRECTION ( 'NONE',  ( -0.000000000000000000, -1.000000000000000000, -0.000000000000000000 ) ) ;
#3315=CIRCLE ( 'NONE', #1965, 7.500000000000007105 ) ;
#3320=CARTESIAN_POINT ( 'NONE',  ( 1.249585401188644101E-12, -6.000000000000005329, -6.421356237309495008 ) ) ;
#3321=CARTESIAN_POINT ( 'NONE',  ( -45.53315400109751465, 12.00000000000000000, -245.3419396193594650 ) ) ;
#3322=DIRECTION ( 'NONE',  ( 0.000000000000000000, 0.000000000000000000, -1.000000000000000000 ) ) ;
#3330=EDGE_CURVE ( 'NONE', #2282, #9776, #3890, .T. ) ;
#3333=CARTESIAN_POINT ( 'NONE',  ( -35.00000000000000000, 12.00000000000002309, -159.6807709998040252 ) ) ;
#3334=EDGE_CURVE ( 'NONE', #11656, #6719, #12016, .T. ) ;
#3337=VECTOR ( 'NONE', #5544, 1000.000000000000000 ) ;
#3348=EDGE_CURVE ( 'NONE', #2194, #8074, #49, .T. ) ;
#3352=CARTESIAN_POINT ( 'NONE',  ( -35.00000000000000000, 12.00000000000001954, -124.6807709998040110 ) ) ;
#3353=ORIENTED_EDGE ( 'NONE', *, *, #3655, .F. ) ;
#3356=EDGE_LOOP ( 'NONE', ( #11380, #3855 ) ) ;
#3359=ORIENTED_EDGE ( 'NONE', *, *, #1844, .F. ) ;
#3362=EDGE_CURVE ( 'NONE', #9776, #338, #367, .T. ) ;
#3368=FACE_BOUND ( 'NONE', #2347, .T. ) ;
#3369=DIRECTION ( 'NONE',  ( 0.000000000000000000, 0.000000000000000000, 1.000000000000000000 ) ) ;
#3370=ORIENTED_EDGE ( 'NONE', *, *, #4133, .T. ) ;
#3374=CYLINDRICAL_SURFACE ( 'NONE', #11416, 7.500000000000007105 ) ;
#3375=DIRECTION ( 'NONE',  ( -0.000000000000000000, 1.000000000000000000, -0.000000000000000000 ) ) ;
#3380=CARTESIAN_POINT ( 'NONE',  ( 154.5043356068769071, 12.00000000000000000, -94.56666130601712439 ) ) ;
#3387=DIRECTION ( 'NONE',  ( -0.000000000000000000, -1.000000000000000000, -0.000000000000000000 ) ) ;
#3388=DIRECTION ( 'NONE',  ( 0.000000000000000000, 0.000000000000000000, -1.000000000000000000 ) ) ;
#3398=VERTEX_POINT ( 'NONE', #1118 ) ;
#3403=AXIS2_PLACEMENT_3D ( 'NONE', #8452, #8557, #9363 ) ;
#3404=CYLINDRICAL_SURFACE ( 'NONE', #7837, 7.500000000000007105 ) ;
#3405=EDGE_CURVE ( 'NONE', #6750, #6717, #5858, .T. ) ;
#3408=CARTESIAN_POINT ( 'NONE',  ( -120.8820948793972434, 12.00000000000000000, -186.6989091883324363 ) ) ;
#3412=ORIENTED_EDGE ( 'NONE', *, *, #1545, .T. ) ;
#3417=CARTESIAN_POINT ( 'NONE',  ( 154.5043356068769071, 0.000000000000000000, -109.5666613060171670 ) ) ;
#3418=VERTEX_POINT ( 'NONE', #7782 ) ;
#3425=CYLINDRICAL_SURFACE ( 'NONE', #3780, 7.500000000000007105 ) ;
#3427=CIRCLE ( 'NONE', #7996, 7.500000000000007105 ) ;
#3428=CARTESIAN_POINT ( 'NONE',  ( 6.257111856936825515E-13, 0.000000000000000000, -73.92135623730949590 ) ) ;
#3430=ADVANCED_FACE ( 'NONE', ( #6672 ), #168, .F. ) ;
#3440=AXIS2_PLACEMENT_3D ( 'NONE', #4510, #3559, #12128 ) ;
#3441=CARTESIAN_POINT ( 'NONE',  ( 2.186774452080127126E-12, 12.00000000000000000, 91.07864376269050410 ) ) ;
#3443=CARTESIAN_POINT ( 'NONE',  ( 151.3258811035896656, 0.000000000000000000, -56.13263083939798292 ) ) ;
#3451=FACE_BOUND ( 'NONE', #10289, .T. ) ;
#3453=DIRECTION ( 'NONE',  ( -0.000000000000000000, 1.000000000000000000, -0.000000000000000000 ) ) ;
#3454=ORIENTED_EDGE ( 'NONE', *, *, #8431, .T. ) ;
#3463=CARTESIAN_POINT ( 'NONE',  ( 1.387778780781445676E-14, 11.99999999999999645, 126.4213562373094959 ) ) ;
#3465=ORIENTED_EDGE ( 'NONE', *, *, #5532, .T. ) ;
#3469=DIRECTION ( 'NONE',  ( 0.000000000000000000, 0.000000000000000000, 1.000000000000000000 ) ) ;
#3472=CARTESIAN_POINT ( 'NONE',  ( 9.184850993605161750E-16, 164.0000000000000000, -133.9213562373095101 ) ) ;
#3473=CIRCLE ( 'NONE', #1915, 7.500000000000007994 ) ;
#3481=LINE ( 'NONE', #7267, #1291 ) ;
#3485=EDGE_CURVE ( 'NONE', #8074, #7241, #9042, .T. ) ;
#3488=DIRECTION ( 'NONE',  ( 0.000000000000000000, 0.000000000000000000, -1.000000000000000000 ) ) ;
#3493=ORIENTED_EDGE ( 'NONE', *, *, #8467, .F. ) ;
#3498=CARTESIAN_POINT ( 'NONE',  ( 1.479627290717497352E-14, 0.000000000000000000, 118.9213562373094817 ) ) ;
#3499=CARTESIAN_POINT ( 'NONE',  ( 1.387778780781445676E-14, 152.0000000000000284, 126.4213562373094959 ) ) ;
#3500=DIRECTION ( 'NONE',  ( 0.000000000000000000, 0.000000000000000000, 1.000000000000000000 ) ) ;
#3501=EDGE_CURVE ( 'NONE', #4515, #3716, #1469, .T. ) ;
#3506=CARTESIAN_POINT ( 'NONE',  ( -45.53315400109751465, 12.00000000000000000, -237.8419396193594650 ) ) ;
#3512=CARTESIAN_POINT ( 'NONE',  ( 3.123963502971610252E-13, -6.000000000000005329, -96.42135623730949590 ) ) ;
#3513=ORIENTED_EDGE ( 'NONE', *, *, #11610, .T. ) ;
#3514=CYLINDRICAL_SURFACE ( 'NONE', #8967, 7.499999999999978684 ) ;
#3516=SURFACE_SIDE_STYLE ('',( #3574 ) ) ;
#3517=EDGE_LOOP ( 'NONE', ( #3003, #998, #2416, #8891 ) ) ;
#3521=AXIS2_PLACEMENT_3D ( 'NONE', #11431, #10562, #11624 ) ;
#3525=ORIENTED_EDGE ( 'NONE', *, *, #6062, .T. ) ;
#3537=ORIENTED_EDGE ( 'NONE', *, *, #2465, .F. ) ;
#3538=FACE_BOUND ( 'NONE', #9519, .T. ) ;
#3540=ORIENTED_EDGE ( 'NONE', *, *, #2286, .F. ) ;
#3545=LINE ( 'NONE', #11106, #5160 ) ;
#3546=ADVANCED_FACE ( 'NONE', ( #5049 ), #7032, .F. ) ;
#3558=CARTESIAN_POINT ( 'NONE',  ( 6.247927005943220505E-13, 12.00000000000000000, -58.92135623730948879 ) ) ;
#3559=DIRECTION ( 'NONE',  ( 0.000000000000000000, 1.000000000000000000, 0.000000000000000000 ) ) ;
#3561=VERTEX_POINT ( 'NONE', #2341 ) ;
#3564=LINE ( 'NONE', #875, #6753 ) ;
#3565=CARTESIAN_POINT ( 'NONE',  ( 1.387778780781445676E-14, -58.00000000000000711, 133.9213562373095101 ) ) ;
#3569=CARTESIAN_POINT ( 'NONE',  ( 0.000000000000000000, -58.00000000000000711, -118.9213562373094817 ) ) ;
#3574=SURFACE_STYLE_FILL_AREA ( #2362 ) ;
#3580=ORIENTED_EDGE ( 'NONE', *, *, #7508, .T. ) ;
#3584=EDGE_CURVE ( 'NONE', #4959, #8782, #4127, .T. ) ;
#3591=VERTEX_POINT ( 'NONE', #9998 ) ;
#3594=CARTESIAN_POINT ( 'NONE',  ( 9.184850993605161750E-16, 11.99999999999999645, -133.9213562373095101 ) ) ;
#3597=CARTESIAN_POINT ( 'NONE',  ( 6.247927005943220505E-13, 164.0000000000000000, -66.42135623730948168 ) ) ;
#3599=DIRECTION ( 'NONE',  ( 0.000000000000000000, 1.000000000000000000, 0.000000000000000000 ) ) ;
#3600=DIRECTION ( 'NONE',  ( 0.000000000000000000, 0.000000000000000000, 1.000000000000000000 ) ) ;
#3606=CARTESIAN_POINT ( 'NONE',  ( 0.000000000000000000, 12.00000000000000000, -89.68077099980401101 ) ) ;
#3608=VECTOR ( 'NONE', #11555, 1000.000000000000000 ) ;
#3609=CARTESIAN_POINT ( 'NONE',  ( -6.106226635438360972E-13, 12.00000000000000000, -252.1807709998039115 ) ) ;
#3611=CARTESIAN_POINT ( 'NONE',  ( -126.4213562373094959, 0.000000000000000000, 2.255140518769849223E-14 ) ) ;
#3615=VECTOR ( 'NONE', #6875, 1000.000000000000000 ) ;
#3621=ORIENTED_EDGE ( 'NONE', *, *, #1457, .F. ) ;
#3626=CARTESIAN_POINT ( 'NONE',  ( -154.5043356068770493, 0.000000000000000000, -109.5666613060160586 ) ) ;
#3627=AXIS2_PLACEMENT_3D ( 'NONE', #4275, #550, #8101 ) ;
#3628=AXIS2_PLACEMENT_3D ( 'NONE', #2437, #519, #5337 ) ;
#3629=VECTOR ( 'NONE', #7890, 1000.000000000000000 ) ;
#3635=DIRECTION ( 'NONE',  ( 0.000000000000000000, 0.000000000000000000, -1.000000000000000000 ) ) ;
#3637=AXIS2_PLACEMENT_3D ( 'NONE', #4591, #1065, #4940 ) ;
#3639=DIRECTION ( 'NONE',  ( -0.000000000000000000, -1.000000000000000000, -0.000000000000000000 ) ) ;
#3640=AXIS2_PLACEMENT_3D ( 'NONE', #736, #9264, #806 ) ;
#3647=EDGE_LOOP ( 'NONE', ( #5089, #5481, #1564, #9524, #10935 ) ) ;
#3652=CIRCLE ( 'NONE', #5223, 7.500000000000020428 ) ;
#3653=AXIS2_PLACEMENT_3D ( 'NONE', #7081, #11899, #2383 ) ;
#3654=EDGE_LOOP ( 'NONE', ( #4821, #4784, #3184, #7823 ) ) ;
#3655=EDGE_CURVE ( 'NONE', #9404, #2620, #1429, .T. ) ;
#3658=ORIENTED_EDGE ( 'NONE', *, *, #6321, .F. ) ;
#3661=CARTESIAN_POINT ( 'NONE',  ( 154.5043356068769071, 0.000000000000000000, -102.0666613060171386 ) ) ;
#3663=CARTESIAN_POINT ( 'NONE',  ( 0.000000000000000000, 12.00000000000000000, -264.6807709998040536 ) ) ;
#3675=AXIS2_PLACEMENT_3D ( 'NONE', #10883, #7934, #3221 ) ;
#3676=ORIENTED_EDGE ( 'NONE', *, *, #9653, .T. ) ;
#3679=VERTEX_POINT ( 'NONE', #4096 ) ;
#3684=AXIS2_PLACEMENT_3D ( 'NONE', #7324, #11026, #11155 ) ;
#3694=CIRCLE ( 'NONE', #9224, 7.500000000000007105 ) ;
#3697=DIRECTION ( 'NONE',  ( 0.000000000000000000, 0.000000000000000000, 1.000000000000000000 ) ) ;
#3702=ORIENTED_EDGE ( 'NONE', *, *, #7352, .F. ) ;
#3703=CARTESIAN_POINT ( 'NONE',  ( 1.387778780781445676E-14, -58.00000000000000711, 126.4213562373094959 ) ) ;
#3707=DIRECTION ( 'NONE',  ( 0.000000000000000000, -1.189524669241239115E-16, 1.000000000000000000 ) ) ;
#3711=DIRECTION ( 'NONE',  ( -0.000000000000000000, 1.000000000000000000, 7.930164461608263644E-17 ) ) ;
#3714=ORIENTED_EDGE ( 'NONE', *, *, #10976, .F. ) ;
#3716=VERTEX_POINT ( 'NONE', #7926 ) ;
#3720=EDGE_CURVE ( 'NONE', #2170, #5214, #3923, .T. ) ;
#3723=CARTESIAN_POINT ( 'NONE',  ( 6.247927005943220505E-13, 0.000000000000000000, -66.42135623730949590 ) ) ;
#3729=CYLINDRICAL_SURFACE ( 'NONE', #11609, 7.500000000000007105 ) ;
#3730=AXIS2_PLACEMENT_3D ( 'NONE', #7218, #1297, #10923 ) ;
#3731=CIRCLE ( 'NONE', #12217, 175.0000000000000000 ) ;
#3734=DIRECTION ( 'NONE',  ( -0.000000000000000000, -1.000000000000000000, -0.000000000000000000 ) ) ;
#3741=FACE_BOUND ( 'NONE', #798, .T. ) ;
#3744=VERTEX_POINT ( 'NONE', #554 ) ;
#3747=AXIS2_PLACEMENT_3D ( 'NONE', #5667, #11353, #1967 ) ;
#3749=CARTESIAN_POINT ( 'NONE',  ( -154.5043356068770493, 12.00000000000000000, -102.0666613060160302 ) ) ;
#3755=EDGE_CURVE ( 'NONE', #10145, #4307, #10832, .T. ) ;
#3756=EDGE_LOOP ( 'NONE', ( #7145, #8148, #2298, #9289 ) ) ;
#3764=CARTESIAN_POINT ( 'NONE',  ( -120.8820948793972434, 0.000000000000000000, -186.6989091883324363 ) ) ;
#3770=CARTESIAN_POINT ( 'NONE',  ( -144.0488662551579182, 0.000000000000000000, -154.4077238332691877 ) ) ;
#3771=CARTESIAN_POINT ( 'NONE',  ( 9.184850993605161750E-16, 152.0000000000000284, -133.9213562373095101 ) ) ;
#3772=ORIENTED_EDGE ( 'NONE', *, *, #253, .T. ) ;
#3774=ORIENTED_EDGE ( 'NONE', *, *, #8809, .F. ) ;
#3776=LINE ( 'NONE', #5003, #1618 ) ;
#3780=AXIS2_PLACEMENT_3D ( 'NONE', #5345, #1522, #8085 ) ;
#3786=DIRECTION ( 'NONE',  ( -0.000000000000000000, -1.000000000000000000, -0.000000000000000000 ) ) ;
#3790=DIRECTION ( 'NONE',  ( 0.000000000000000000, -1.156482317317870246E-16, 1.000000000000000000 ) ) ;
#3796=AXIS2_PLACEMENT_3D ( 'NONE', #8383, #5519, #834 ) ;
#3804=CARTESIAN_POINT ( 'NONE',  ( 35.00000000000000000, 163.9999999999999716, 190.3192290001959748 ) ) ;
#3805=CYLINDRICAL_SURFACE ( 'NONE', #7967, 35.00000000000002842 ) ;
#3806=DIRECTION ( 'NONE',  ( 0.000000000000000000, 1.000000000000000000, 0.000000000000000000 ) ) ;
#3808=PRODUCT_DEFINITION_CONTEXT ( 'detailed design', #9041, 'design' ) ;
#3812=VERTEX_POINT ( 'NONE', #1603 ) ;
#3817=CARTESIAN_POINT ( 'NONE',  ( 35.00000000000000000, 12.00000000000000000, 40.70327710424895429 ) ) ;
#3820=EDGE_CURVE ( 'NONE', #9670, #5146, #7293, .T. ) ;
#3828=EDGE_CURVE ( 'NONE', #4476, #7628, #4136, .T. ) ;
#3834=CIRCLE ( 'NONE', #7584, 7.500000000000007105 ) ;
#3835=CIRCLE ( 'NONE', #1086, 81.99999999999998579 ) ;
#3840=EDGE_LOOP ( 'NONE', ( #10910, #3537 ) ) ;
#3844=AXIS2_PLACEMENT_3D ( 'NONE', #6142, #640, #7258 ) ;
#3847=ORIENTED_EDGE ( 'NONE', *, *, #2427, .T. ) ;
#3852=ORIENTED_EDGE ( 'NONE', *, *, #3348, .T. ) ;
#3855=ORIENTED_EDGE ( 'NONE', *, *, #6665, .T. ) ;
#3867=ORIENTED_EDGE ( 'NONE', *, *, #7290, .T. ) ;
#3871=DIRECTION ( 'NONE',  ( 0.000000000000000000, -1.156482317317870246E-16, 1.000000000000000000 ) ) ;
#3876=EDGE_LOOP ( 'NONE', ( #3227, #1674 ) ) ;
#3877=EDGE_CURVE ( 'NONE', #3054, #8695, #2751, .T. ) ;
#3881=VECTOR ( 'NONE', #3786, 1000.000000000000000 ) ;
#3890=LINE ( 'NONE', #4991, #1759 ) ;
#3895=DIRECTION ( 'NONE',  ( -0.000000000000000000, -1.000000000000000000, -0.000000000000000000 ) ) ;
#3897=CIRCLE ( 'NONE', #8453, 7.500000000000020428 ) ;
#3898=FACE_BOUND ( 'NONE', #3938, .T. ) ;
#3909=DIRECTION ( 'NONE',  ( -0.000000000000000000, -1.000000000000000000, -0.000000000000000000 ) ) ;
#3915=AXIS2_PLACEMENT_3D ( 'NONE', #2250, #8118, #11883 ) ;
#3919=CARTESIAN_POINT ( 'NONE',  ( 9.381075359908434252E-13, -6.000000000000004441, -43.92135623730950300 ) ) ;
#3923=CIRCLE ( 'NONE', #5498, 7.500000000000007105 ) ;
#3927=EDGE_LOOP ( 'NONE', ( #3676, #315, #2634, #4068 ) ) ;
#3928=AXIS2_PLACEMENT_3D ( 'NONE', #285, #7711, #1173 ) ;
#3930=ORIENTED_EDGE ( 'NONE', *, *, #3053, .T. ) ;
#3932=DIRECTION ( 'NONE',  ( -0.000000000000000000, -1.000000000000000000, -0.000000000000000000 ) ) ;
#3938=EDGE_LOOP ( 'NONE', ( #2981, #3105 ) ) ;
#3944=LINE ( 'NONE', #2959, #4523 ) ;
#3948=DIRECTION ( 'NONE',  ( 0.000000000000000000, 1.000000000000000000, 0.000000000000000000 ) ) ;
#3950=CARTESIAN_POINT ( 'NONE',  ( -144.0488662551579182, 12.00000000000000000, -146.9077238332691877 ) ) ;
#3953=CARTESIAN_POINT ( 'NONE',  ( 0.000000000000000000, 0.000000000000000000, -89.68077099980401101 ) ) ;
#3954=ORIENTED_EDGE ( 'NONE', *, *, #3181, .T. ) ;
#3958=FACE_BOUND ( 'NONE', #4353, .T. ) ;
#3966=ORIENTED_EDGE ( 'NONE', *, *, #2818, .F. ) ;
#3972=AXIS2_PLACEMENT_3D ( 'NONE', #11664, #8069, #1510 ) ;
#3973=ORIENTED_EDGE ( 'NONE', *, *, #6074, .T. ) ;
#3975=ORIENTED_EDGE ( 'NONE', *, *, #5169, .F. ) ;
#3976=EDGE_CURVE ( 'NONE', #3716, #1640, #9463, .T. ) ;
#3981=CARTESIAN_POINT ( 'NONE',  ( 9.371890508914830252E-13, 0.000000000000000000, -36.42135623730949590 ) ) ;
#3985=EDGE_LOOP ( 'NONE', ( #7495, #685, #4363, #6562 ) ) ;
#3991=VECTOR ( 'NONE', #5112, 1000.000000000000000 ) ;
#3993=DIRECTION ( 'NONE',  ( 0.000000000000000000, -1.156482317317870246E-16, 1.000000000000000000 ) ) ;
#3995=EDGE_CURVE ( 'NONE', #1396, #6687, #6172, .T. ) ;
#4000=AXIS2_PLACEMENT_3D ( 'NONE', #8837, #10865, #3206 ) ;
#4005=ORIENTED_EDGE ( 'NONE', *, *, #8930, .T. ) ;
#4012=DIRECTION ( 'NONE',  ( -0.000000000000000000, 1.000000000000000000, 7.930164461608263644E-17 ) ) ;
#4017=DIRECTION ( 'NONE',  ( 0.000000000000000000, 0.000000000000000000, 1.000000000000000000 ) ) ;
#4024=VECTOR ( 'NONE', #1889, 1000.000000000000000 ) ;
#4025=DIRECTION ( 'NONE',  ( 0.000000000000000000, 1.000000000000000000, 0.000000000000000000 ) ) ;
#4029=DIRECTION ( 'NONE',  ( 0.000000000000000000, 0.000000000000000000, 1.000000000000000000 ) ) ;
#4033=EDGE_CURVE ( 'NONE', #5323, #9863, #7092, .T. ) ;
#4038=FACE_OUTER_BOUND ( 'NONE', #6376, .T. ) ;
#4043=ORIENTED_EDGE ( 'NONE', *, *, #789, .T. ) ;
#4045=CIRCLE ( 'NONE', #895, 81.99999999999998579 ) ;
#4049=ORIENTED_EDGE ( 'NONE', *, *, #6369, .T. ) ;
#4052=VERTEX_POINT ( 'NONE', #4141 ) ;
#4053=CIRCLE ( 'NONE', #1886, 134.9999999999999716 ) ;
#4060=CYLINDRICAL_SURFACE ( 'NONE', #7553, 7.500000000000007105 ) ;
#4064=DIRECTION ( 'NONE',  ( 0.000000000000000000, -1.156482317317870246E-16, 1.000000000000000000 ) ) ;
#4068=ORIENTED_EDGE ( 'NONE', *, *, #8952, .F. ) ;
#4073=FACE_OUTER_BOUND ( 'NONE', #1930, .T. ) ;
#4076=ORIENTED_EDGE ( 'NONE', *, *, #5169, .T. ) ;
#4077=CARTESIAN_POINT ( 'NONE',  ( 1.249585401188644101E-12, 164.0000000000000000, -6.421356237309481685 ) ) ;
#4084=CARTESIAN_POINT ( 'NONE',  ( 2.186774452080127126E-12, 12.00000000000000000, 83.57864376269050410 ) ) ;
#4085=DIRECTION ( 'NONE',  ( 0.000000000000000000, 0.000000000000000000, -1.000000000000000000 ) ) ;
#4087=CARTESIAN_POINT ( 'NONE',  ( -144.0488662551579182, 0.000000000000000000, -146.9077238332691877 ) ) ;
#4090=VERTEX_POINT ( 'NONE', #7003 ) ;
#4091=AXIS2_PLACEMENT_3D ( 'NONE', #12015, #8390, #1694 ) ;
#4093=ORIENTED_EDGE ( 'NONE', *, *, #10852, .T. ) ;
#4096=CARTESIAN_POINT ( 'NONE',  ( 1.875296586882326249E-12, 163.9999999999999716, 46.07864376269051121 ) ) ;
#4107=CARTESIAN_POINT ( 'NONE',  ( 126.4213562373094959, 12.00000000000000000, 7.500000000000007105 ) ) ;
#4118=CARTESIAN_POINT ( 'NONE',  ( 1.249585401188644101E-12, 12.00000000000000000, -6.421356237309494119 ) ) ;
#4122=DIRECTION ( 'NONE',  ( 0.000000000000000000, 0.000000000000000000, 1.000000000000000000 ) ) ;
#4127=CIRCLE ( 'NONE', #8284, 7.500000000000007105 ) ;
#4133=EDGE_CURVE ( 'NONE', #9567, #11989, #7063, .T. ) ;
#4136=CIRCLE ( 'NONE', #10644, 7.500000000000007105 ) ;
#4141=CARTESIAN_POINT ( 'NONE',  ( 9.371890508914830252E-13, 164.0000000000000000, -28.92135623730947458 ) ) ;
#4146=CARTESIAN_POINT ( 'NONE',  ( 0.000000000000000000, 12.00000000000000000, -124.6807709998040110 ) ) ;
#4148=ORIENTED_EDGE ( 'NONE', *, *, #8792, .F. ) ;
#4156=DIRECTION ( 'NONE',  ( -0.000000000000000000, -1.000000000000000000, -0.000000000000000000 ) ) ;
#4167=ORIENTED_EDGE ( 'NONE', *, *, #4362, .F. ) ;
#4168=ADVANCED_FACE ( 'NONE', ( #11499 ), #117, .F. ) ;
#4173=DIRECTION ( 'NONE',  ( 0.000000000000000000, 0.000000000000000000, -1.000000000000000000 ) ) ;
#4174=ORIENTED_EDGE ( 'NONE', *, *, #7577, .F. ) ;
#4175=DIRECTION ( 'NONE',  ( 0.000000000000000000, -1.156482317317870246E-16, 1.000000000000000000 ) ) ;
#4177=VECTOR ( 'NONE', #3260, 1000.000000000000000 ) ;
#4187=ADVANCED_FACE ( 'NONE', ( #6039 ), #1401, .F. ) ;
#4198=CIRCLE ( 'NONE', #11706, 7.500000000000013323 ) ;
#4200=CYLINDRICAL_SURFACE ( 'NONE', #10096, 7.500000000000007105 ) ;
#4204=ORIENTED_EDGE ( 'NONE', *, *, #5019, .F. ) ;
#4213=CIRCLE ( 'NONE', #1254, 7.500000000000013323 ) ;
#4219=VECTOR ( 'NONE', #3707, 1000.000000000000000 ) ;
#4224=ORIENTED_EDGE ( 'NONE', *, *, #6619, .T. ) ;
#4228=VECTOR ( 'NONE', #9157, 1000.000000000000000 ) ;
#4234=LINE ( 'NONE', #1020, #6782 ) ;
#4237=DIRECTION ( 'NONE',  ( 0.000000000000000000, 1.000000000000000000, 0.000000000000000000 ) ) ;
#4240=EDGE_LOOP ( 'NONE', ( #3930, #12072 ) ) ;
#4241=AXIS2_PLACEMENT_3D ( 'NONE', #10204, #11934, #10136 ) ;
#4248=EDGE_LOOP ( 'NONE', ( #7773, #7279 ) ) ;
#4255=VECTOR ( 'NONE', #11323, 1000.000000000000000 ) ;
#4257=CIRCLE ( 'NONE', #7402, 7.500000000000007105 ) ;
#4258=EDGE_CURVE ( 'NONE', #11998, #8531, #2043, .T. ) ;
#4261=FACE_BOUND ( 'NONE', #8800, .T. ) ;
#4262=DIRECTION ( 'NONE',  ( 0.000000000000000000, 1.000000000000000000, 0.000000000000000000 ) ) ;
#4264=AXIS2_PLACEMENT_3D ( 'NONE', #1639, #5277, #9051 ) ;
#4266=EDGE_LOOP ( 'NONE', ( #2422, #4697, #5199, #3265 ) ) ;
#4268=DIRECTION ( 'NONE',  ( 0.000000000000000000, 0.000000000000000000, -1.000000000000000000 ) ) ;
#4272=CYLINDRICAL_SURFACE ( 'NONE', #4971, 81.99999999999998579 ) ;
#4273=EDGE_LOOP ( 'NONE', ( #6438, #1483 ) ) ;
#4275=CARTESIAN_POINT ( 'NONE',  ( 3.123963502971610252E-13, 164.0000000000000000, -96.42135623730948168 ) ) ;
#4276=EDGE_CURVE ( 'NONE', #725, #739, #10233, .T. ) ;
#4279=LINE ( 'NONE', #5312, #5478 ) ;
#4285=VERTEX_POINT ( 'NONE', #8021 ) ;
#4288=VERTEX_POINT ( 'NONE', #1458 ) ;
#4289=AXIS2_PLACEMENT_3D ( 'NONE', #10496, #8648, #6721 ) ;
#4301=ORIENTED_EDGE ( 'NONE', *, *, #11364, .F. ) ;
#4306=DIRECTION ( 'NONE',  ( 0.000000000000000000, 1.000000000000000000, 0.000000000000000000 ) ) ;
#4307=VERTEX_POINT ( 'NONE', #525 ) ;
#4312=MECHANICAL_DESIGN_GEOMETRIC_PRESENTATION_REPRESENTATION('',(#4897),#11232);
#4313=CARTESIAN_POINT ( 'NONE',  ( 6.257111856936825515E-13, 152.0000000000000000, -73.92135623730948168 ) ) ;
#4315=FACE_BOUND ( 'NONE', #7098, .T. ) ;
#4325=DIRECTION ( 'NONE',  ( 0.000000000000000000, 0.000000000000000000, 1.000000000000000000 ) ) ;
#4326=CARTESIAN_POINT ( 'NONE',  ( 120.8820948793965186, 12.00000000000000000, -179.1989091883332890 ) ) ;
#4327=ORIENTED_EDGE ( 'NONE', *, *, #10098, .T. ) ;
#4328=AXIS2_PLACEMENT_3D ( 'NONE', #5366, #9142, #8234 ) ;
#4340=ORIENTED_EDGE ( 'NONE', *, *, #9875, .F. ) ;
#4352=ORIENTED_EDGE ( 'NONE', *, *, #10394, .T. ) ;
#4353=EDGE_LOOP ( 'NONE', ( #3154, #11847 ) ) ;
#4355=DIRECTION ( 'NONE',  ( 0.000000000000000000, 1.000000000000000000, 0.000000000000000000 ) ) ;
#4356=EDGE_CURVE ( 'NONE', #4489, #1654, #4494, .T. ) ;
#4362=EDGE_CURVE ( 'NONE', #5569, #8440, #12099, .T. ) ;
#4363=ORIENTED_EDGE ( 'NONE', *, *, #7212, .F. ) ;
#4369=EDGE_CURVE ( 'NONE', #10481, #6037, #9056, .T. ) ;
#4370=CARTESIAN_POINT ( 'NONE',  ( 1.874378101782966050E-12, 0.000000000000000000, 61.07864376269051121 ) ) ;
#4371=CYLINDRICAL_SURFACE ( 'NONE', #2555, 81.99999999999998579 ) ;
#4373=FACE_OUTER_BOUND ( 'NONE', #2372, .T. ) ;
#4374=CARTESIAN_POINT ( 'NONE',  ( 1.249585401188644101E-12, -6.000000000000006217, 1.078643762690512986 ) ) ;
#4380=CARTESIAN_POINT ( 'NONE',  ( 154.5043356068769071, 12.00000000000000000, -109.5666613060171670 ) ) ;
#4387=DIRECTION ( 'NONE',  ( 0.000000000000000000, 0.000000000000000000, -1.000000000000000000 ) ) ;
#4391=CIRCLE ( 'NONE', #9526, 7.500000000000007105 ) ;
#4392=CARTESIAN_POINT ( 'NONE',  ( 6.247927005943220505E-13, -6.000000000000005329, -66.42135623730949590 ) ) ;
#4393=ORIENTED_EDGE ( 'NONE', *, *, #3501, .F. ) ;
#4396=EDGE_LOOP ( 'NONE', ( #7406, #10772 ) ) ;
#4399=EDGE_LOOP ( 'NONE', ( #12050, #5987 ) ) ;
#4403=DIRECTION ( 'NONE',  ( 0.000000000000000000, 1.000000000000000000, 0.000000000000000000 ) ) ;
#4406=CIRCLE ( 'NONE', #11318, 7.500000000000007105 ) ;
#4411=ORIENTED_EDGE ( 'NONE', *, *, #7892, .T. ) ;
#4421=EDGE_LOOP ( 'NONE', ( #5251, #7757, #2175, #1265 ) ) ;
#4422=AXIS2_PLACEMENT_3D ( 'NONE', #3723, #762, #8444 ) ;
#4428=ORIENTED_EDGE ( 'NONE', *, *, #5184, .T. ) ;
#4434=DIRECTION ( 'NONE',  ( -0.000000000000000000, 1.000000000000000000, 7.930164461608263644E-17 ) ) ;
#4439=EDGE_CURVE ( 'NONE', #931, #5557, #6469, .T. ) ;
#4447=DIRECTION ( 'NONE',  ( -0.000000000000000000, 1.000000000000000000, 7.930164461608263644E-17 ) ) ;
#4451=ORIENTED_EDGE ( 'NONE', *, *, #6855, .T. ) ;
#4456=CARTESIAN_POINT ( 'NONE',  ( 144.0488662551573782, 12.00000000000000000, -154.4077238332702393 ) ) ;
#4458=CARTESIAN_POINT ( 'NONE',  ( -87.04832655144203102, 12.00000000000000000, -225.4289243767377116 ) ) ;
#4462=DIRECTION ( 'NONE',  ( -0.000000000000000000, 1.000000000000000000, 7.930164461608263644E-17 ) ) ;
#4463=VERTEX_POINT ( 'NONE', #7334 ) ;
#4466=CIRCLE ( 'NONE', #11368, 7.500000000000007105 ) ;
#4468=ORIENTED_EDGE ( 'NONE', *, *, #9777, .F. ) ;
#4471=VERTEX_POINT ( 'NONE', #11102 ) ;
#4476=VERTEX_POINT ( 'NONE', #6404 ) ;
#4478=EDGE_CURVE ( 'NONE', #1936, #2170, #5471, .T. ) ;
#4483=LINE ( 'NONE', #8257, #3293 ) ;
#4484=AXIS2_PLACEMENT_3D ( 'NONE', #1631, #10345, #10285 ) ;
#4486=CARTESIAN_POINT ( 'NONE',  ( 1.874378101782966050E-12, 12.00000000000000000, 53.57864376269050410 ) ) ;
#4488=SHAPE_REPRESENTATION ( 'Bending Angle Gauge Plate', ( #11957 ), #6826 ) ;
#4489=VERTEX_POINT ( 'NONE', #9495 ) ;
#4494=LINE ( 'NONE', #3609, #10624 ) ;
#4498=DIRECTION ( 'NONE',  ( 0.000000000000000000, -1.000000000000000000, -2.312964634635740689E-15 ) ) ;
#4506=ORIENTED_EDGE ( 'NONE', *, *, #4439, .F. ) ;
#4509=CARTESIAN_POINT ( 'NONE',  ( 3.123963502971610252E-13, -6.000000000000005329, -96.42135623730949590 ) ) ;
#4510=CARTESIAN_POINT ( 'NONE',  ( 151.3258811035896656, 0.000000000000000000, -56.13263083939798292 ) ) ;
#4515=VERTEX_POINT ( 'NONE', #920 ) ;
#4523=VECTOR ( 'NONE', #6722, 1000.000000000000000 ) ;
#4529=LINE ( 'NONE', #6367, #1955 ) ;
#4531=ORIENTED_EDGE ( 'NONE', *, *, #2299, .T. ) ;
#4532=CARTESIAN_POINT ( 'NONE',  ( -120.8820948793972434, 12.00000000000000000, -194.1989091883324363 ) ) ;
#4536=ORIENTED_EDGE ( 'NONE', *, *, #9981, .T. ) ;
#4541=CARTESIAN_POINT ( 'NONE',  ( -126.4213562373094959, 12.00000000000000000, 2.255140518769849223E-14 ) ) ;
#4545=CARTESIAN_POINT ( 'NONE',  ( 2.186774452080127126E-12, 0.000000000000000000, 83.57864376269050410 ) ) ;
#4549=DIRECTION ( 'NONE',  ( 0.000000000000000000, 1.000000000000000000, 0.000000000000000000 ) ) ;
#4550=CARTESIAN_POINT ( 'NONE',  ( 6.257111856936825515E-13, 164.0000000000000000, -73.92135623730948168 ) ) ;
#4553=VERTEX_POINT ( 'NONE', #4800 ) ;
#4554=FACE_BOUND ( 'NONE', #8597, .T. ) ;
#4556=ORIENTED_EDGE ( 'NONE', *, *, #10469, .T. ) ;
#4557=CARTESIAN_POINT ( 'NONE',  ( 144.0488662551573782, 12.00000000000000000, -146.9077238332702109 ) ) ;
#4561=DIRECTION ( 'NONE',  ( -0.000000000000000000, 1.000000000000000000, -0.000000000000000000 ) ) ;
#4566=ORIENTED_EDGE ( 'NONE', *, *, #6321, .T. ) ;
#4567=ORIENTED_EDGE ( 'NONE', *, *, #6967, .F. ) ;
#4575=AXIS2_PLACEMENT_3D ( 'NONE', #4917, #215, #4064 ) ;
#4577=DIRECTION ( 'NONE',  ( 0.000000000000000000, 0.000000000000000000, 1.000000000000000000 ) ) ;
#4578=CYLINDRICAL_SURFACE ( 'NONE', #6419, 7.500000000000007105 ) ;
#4582=EDGE_LOOP ( 'NONE', ( #1503, #3966 ) ) ;
#4586=CARTESIAN_POINT ( 'NONE',  ( 9.371890508914830252E-13, 164.0000000000000000, -36.42135623730948168 ) ) ;
#4591=CARTESIAN_POINT ( 'NONE',  ( 6.247927005943220505E-13, -6.000000000000005329, -66.42135623730949590 ) ) ;
#4601=VERTEX_POINT ( 'NONE', #7641 ) ;
#4602=VECTOR ( 'NONE', #6982, 1000.000000000000000 ) ;
#4605=VERTEX_POINT ( 'NONE', #3804 ) ;
#4610=VECTOR ( 'NONE', #1382, 1000.000000000000000 ) ;
#4622=ADVANCED_FACE ( 'NONE', ( #10483 ), #4852, .F. ) ;
#4627=DIRECTION ( 'NONE',  ( 0.000000000000000000, 1.000000000000000000, 0.000000000000000000 ) ) ;
#4639=CARTESIAN_POINT ( 'NONE',  ( 2.187692937179487324E-12, -6.000000000000004441, 76.07864376269048989 ) ) ;
#4640=CIRCLE ( 'NONE', #5607, 7.500000000000013323 ) ;
#4641=ADVANCED_FACE ( 'NONE', ( #6766 ), #8697, .F. ) ;
#4643=AXIS2_PLACEMENT_3D ( 'NONE', #6767, #6893, #11538 ) ;
#4647=DIRECTION ( 'NONE',  ( -0.000000000000000000, -1.000000000000000000, -0.000000000000000000 ) ) ;
#4648=DIRECTION ( 'NONE',  ( -1.000000000000000000, -0.000000000000000000, -0.000000000000000000 ) ) ;
#4650=AXIS2_PLACEMENT_3D ( 'NONE', #8607, #8546, #6628 ) ;
#4654=DIRECTION ( 'NONE',  ( 0.000000000000000000, 1.000000000000000000, 0.000000000000000000 ) ) ;
#4656=DIRECTION ( 'NONE',  ( 0.000000000000000000, 0.000000000000000000, 1.000000000000000000 ) ) ;
#4666=EDGE_LOOP ( 'NONE', ( #3714, #7552, #1376, #2606 ) ) ;
#4668=DIRECTION ( 'NONE',  ( -0.000000000000000000, 1.000000000000000000, 0.000000000000000000 ) ) ;
#4675=EDGE_CURVE ( 'NONE', #6037, #5102, #6544, .T. ) ;
#4677=DIRECTION ( 'NONE',  ( 0.000000000000000000, 0.000000000000000000, 1.000000000000000000 ) ) ;
#4682=ORIENTED_EDGE ( 'NONE', *, *, #14, .T. ) ;
#4692=AXIS2_PLACEMENT_3D ( 'NONE', #2556, #7259, #7506 ) ;
#4697=ORIENTED_EDGE ( 'NONE', *, *, #8310, .F. ) ;
#4700=ORIENTED_EDGE ( 'NONE', *, *, #2760, .F. ) ;
#4702=ORIENTED_EDGE ( 'NONE', *, *, #8310, .T. ) ;
#4703=AXIS2_PLACEMENT_3D ( 'NONE', #3661, #11331, #901 ) ;
#4708=ADVANCED_FACE ( 'NONE', ( #7088 ), #11732, .F. ) ;
#4714=VERTEX_POINT ( 'NONE', #6163 ) ;
#4720=CIRCLE ( 'NONE', #6094, 7.500000000000007105 ) ;
#4729=AXIS2_PLACEMENT_3D ( 'NONE', #7716, #1180, #2964 ) ;
#4730=ADVANCED_FACE ( 'NONE', ( #2274 ), #1230, .F. ) ;
#4731=DIRECTION ( 'NONE',  ( 0.000000000000000000, 0.000000000000000000, -1.000000000000000000 ) ) ;
#4732=DIRECTION ( 'NONE',  ( 0.000000000000000000, 0.000000000000000000, 1.000000000000000000 ) ) ;
#4736=DIRECTION ( 'NONE',  ( 0.000000000000000000, 1.000000000000000000, 0.000000000000000000 ) ) ;
#4743=CYLINDRICAL_SURFACE ( 'NONE', #8243, 7.500000000000007105 ) ;
#4745=EDGE_CURVE ( 'NONE', #3812, #4910, #11617, .T. ) ;
#4748=EDGE_CURVE ( 'NONE', #3744, #5923, #3249, .T. ) ;
#4749=EDGE_LOOP ( 'NONE', ( #1424, #1005, #10893, #5530 ) ) ;
#4751=VERTEX_POINT ( 'NONE', #6966 ) ;
#4752=EDGE_CURVE ( 'NONE', #3398, #12119, #6042, .T. ) ;
#4756=ORIENTED_EDGE ( 'NONE', *, *, #4258, .F. ) ;
#4757=CARTESIAN_POINT ( 'NONE',  ( -120.8820948793972434, 0.000000000000000000, -186.6989091883324363 ) ) ;
#4758=DIRECTION ( 'NONE',  ( 0.000000000000000000, 0.000000000000000000, 1.000000000000000000 ) ) ;
#4763=DIRECTION ( 'NONE',  ( 0.000000000000000000, -1.156482317317870246E-16, 1.000000000000000000 ) ) ;
#4767=PRODUCT ( 'Bending Angle Gauge Plate', 'Bending Angle Gauge Plate', '', ( #6890 ) ) ;
#4776=DIRECTION ( 'NONE',  ( 0.000000000000000000, 0.000000000000000000, 1.000000000000000000 ) ) ;
#4784=ORIENTED_EDGE ( 'NONE', *, *, #1792, .F. ) ;
#4787=CYLINDRICAL_SURFACE ( 'NONE', #1909, 7.500000000000007994 ) ;
#4789=ADVANCED_FACE ( 'NONE', ( #10981 ), #3425, .F. ) ;
#4792=VERTEX_POINT ( 'NONE', #4370 ) ;
#4798=ORIENTED_EDGE ( 'NONE', *, *, #7505, .F. ) ;
#4800=CARTESIAN_POINT ( 'NONE',  ( -87.04832655144203102, 0.000000000000000000, -210.4289243767376831 ) ) ;
#4801=LINE ( 'NONE', #1100, #3629 ) ;
#4802=CARTESIAN_POINT ( 'NONE',  ( 154.5043356068769071, 0.000000000000000000, -102.0666613060171386 ) ) ;
#4806=FACE_OUTER_BOUND ( 'NONE', #7673, .T. ) ;
#4810=PLANE ( 'NONE',  #5253 ) ;
#4815=ORIENTED_EDGE ( 'NONE', *, *, #8680, .F. ) ;
#4821=ORIENTED_EDGE ( 'NONE', *, *, #6369, .F. ) ;
#4825=FACE_BOUND ( 'NONE', #1576, .T. ) ;
#4827=ORIENTED_EDGE ( 'NONE', *, *, #9479, .T. ) ;
#4828=CIRCLE ( 'NONE', #6407, 7.500000000000007105 ) ;
#4835=LINE ( 'NONE', #131, #9554 ) ;
#4837=DIRECTION ( 'NONE',  ( -1.000000000000000000, -0.000000000000000000, 0.000000000000000000 ) ) ;
#4838=ORIENTED_EDGE ( 'NONE', *, *, #9507, .T. ) ;
#4845=ORIENTED_EDGE ( 'NONE', *, *, #3334, .T. ) ;
#4847=DIRECTION ( 'NONE',  ( 0.000000000000000000, 0.000000000000000000, 1.000000000000000000 ) ) ;
#4848=EDGE_LOOP ( 'NONE', ( #7835, #10364, #3038, #5376 ) ) ;
#4850=ORIENTED_EDGE ( 'NONE', *, *, #5479, .F. ) ;
#4852=CYLINDRICAL_SURFACE ( 'NONE', #11488, 7.500000000000013323 ) ;
#4853=DIRECTION ( 'NONE',  ( 0.000000000000000000, 0.000000000000000000, 1.000000000000000000 ) ) ;
#4862=EDGE_CURVE ( 'NONE', #7231, #4601, #3545, .T. ) ;
#4864=CARTESIAN_POINT ( 'NONE',  ( 144.0488662551573782, 12.00000000000000000, -139.4077238332702109 ) ) ;
#4870=DIRECTION ( 'NONE',  ( 0.000000000000000000, 1.000000000000000000, 0.000000000000000000 ) ) ;
#4873=DIRECTION ( 'NONE',  ( 0.000000000000000000, 1.000000000000000000, 0.000000000000000000 ) ) ;
#4874=DIRECTION ( 'NONE',  ( 0.000000000000000000, 0.000000000000000000, 1.000000000000000000 ) ) ;
#4875=ORIENTED_EDGE ( 'NONE', *, *, #9843, .T. ) ;
#4881=ADVANCED_FACE ( 'NONE', ( #9315 ), #10632, .F. ) ;
#4882=FACE_BOUND ( 'NONE', #11100, .T. ) ;
#4891=CARTESIAN_POINT ( 'NONE',  ( 1.387778780781445676E-14, 11.99999999999999645, 133.9213562373095101 ) ) ;
#4897=STYLED_ITEM ( 'NONE', ( #6252 ), #8194 ) ;
#4899=DIRECTION ( 'NONE',  ( -0.000000000000000000, 1.000000000000000000, 7.930164461608263644E-17 ) ) ;
#4901=CARTESIAN_POINT ( 'NONE',  ( 3.133148353965215262E-13, 152.0000000000000000, -103.9213562373094817 ) ) ;
#4903=ORIENTED_EDGE ( 'NONE', *, *, #199, .T. ) ;
#4907=VERTEX_POINT ( 'NONE', #4999 ) ;
#4910=VERTEX_POINT ( 'NONE', #5934 ) ;
#4917=CARTESIAN_POINT ( 'NONE',  ( 9.371890508914830252E-13, -6.000000000000005329, -36.42135623730949590 ) ) ;
#4919=CARTESIAN_POINT ( 'NONE',  ( 120.8820948793965186, 0.000000000000000000, -186.6989091883332890 ) ) ;
#4927=DIRECTION ( 'NONE',  ( -0.000000000000000000, -1.000000000000000000, -0.000000000000000000 ) ) ;
#4931=FACE_OUTER_BOUND ( 'NONE', #6476, .T. ) ;
#4933=DIRECTION ( 'NONE',  ( 0.000000000000000000, -1.000000000000000000, -7.930164461608263644E-17 ) ) ;
#4939=EDGE_LOOP ( 'NONE', ( #12216, #9649 ) ) ;
#4940=DIRECTION ( 'NONE',  ( 0.000000000000000000, -1.156482317317870246E-16, 1.000000000000000000 ) ) ;
#4942=EDGE_CURVE ( 'NONE', #6687, #3591, #10498, .T. ) ;
#4944=FACE_BOUND ( 'NONE', #1687, .T. ) ;
#4950=FACE_OUTER_BOUND ( 'NONE', #12207, .T. ) ;
#4959=VERTEX_POINT ( 'NONE', #9761 ) ;
#4960=CARTESIAN_POINT ( 'NONE',  ( -120.8820948793972434, 12.00000000000000000, -179.1989091883324363 ) ) ;
#4961=VECTOR ( 'NONE', #9746, 1000.000000000000000 ) ;
#4964=ORIENTED_EDGE ( 'NONE', *, *, #2893, .T. ) ;
#4966=ORIENTED_EDGE ( 'NONE', *, *, #10682, .T. ) ;
#4967=CARTESIAN_POINT ( 'NONE',  ( 0.000000000000000000, 0.000000000000000000, -264.6807709998040536 ) ) ;
#4968=ORIENTED_EDGE ( 'NONE', *, *, #6853, .F. ) ;
#4971=AXIS2_PLACEMENT_3D ( 'NONE', #1363, #8946, #3153 ) ;
#4978=EDGE_LOOP ( 'NONE', ( #4995, #2678, #12060, #11832 ) ) ;
#4980=VERTEX_POINT ( 'NONE', #9886 ) ;
#4985=DIRECTION ( 'NONE',  ( 0.000000000000000000, -1.156482317317870246E-16, 1.000000000000000000 ) ) ;
#4988=CARTESIAN_POINT ( 'NONE',  ( 1.249585401188644101E-12, 164.0000000000000000, 1.078643762690527641 ) ) ;
#4991=CARTESIAN_POINT ( 'NONE',  ( 87.04832655144112152, 12.00000000000000000, -210.4289243767383368 ) ) ;
#4995=ORIENTED_EDGE ( 'NONE', *, *, #8066, .F. ) ;
#4997=CARTESIAN_POINT ( 'NONE',  ( 0.000000000000000000, 164.0000000000000000, -126.4213562373094959 ) ) ;
#4998=ADVANCED_FACE ( 'NONE', ( #2351 ), #4200, .F. ) ;
#4999=CARTESIAN_POINT ( 'NONE',  ( 35.00000000000000000, 2.012279232133096230E-14, -124.6807709998040110 ) ) ;
#5001=CYLINDRICAL_SURFACE ( 'NONE', #97, 7.500000000000007105 ) ;
#5003=CARTESIAN_POINT ( 'NONE',  ( -6.097041784444755962E-13, 12.00000000000000000, -237.1807709998039115 ) ) ;
#5012=ADVANCED_FACE ( 'NONE', ( #11631 ), #10688, .F. ) ;
#5013=CIRCLE ( 'NONE', #9757, 7.500000000000007105 ) ;
#5016=VECTOR ( 'NONE', #8486, 1000.000000000000000 ) ;
#5019=EDGE_CURVE ( 'NONE', #7819, #10381, #6343, .T. ) ;
#5026=DIRECTION ( 'NONE',  ( 0.000000000000000000, 1.000000000000000000, 0.000000000000000000 ) ) ;
#5027=ORIENTED_EDGE ( 'NONE', *, *, #9627, .F. ) ;
#5029=AXIS2_PLACEMENT_3D ( 'NONE', #1386, #4355, #2491 ) ;
#5030=ORIENTED_EDGE ( 'NONE', *, *, #11602, .F. ) ;
#5032=CARTESIAN_POINT ( 'NONE',  ( 1.250503886288004501E-12, 164.0000000000000000, -13.92135623730949057 ) ) ;
#5033=EDGE_CURVE ( 'NONE', #10254, #8307, #11749, .T. ) ;
#5039=DIRECTION ( 'NONE',  ( -0.000000000000000000, 1.000000000000000000, 7.930164461608263644E-17 ) ) ;
#5048=DIRECTION ( 'NONE',  ( 0.000000000000000000, 0.000000000000000000, 1.000000000000000000 ) ) ;
#5049=FACE_OUTER_BOUND ( 'NONE', #75, .T. ) ;
#5054=DIRECTION ( 'NONE',  ( 0.000000000000000000, 1.000000000000000000, 0.000000000000000000 ) ) ;
#5061=AXIS2_PLACEMENT_3D ( 'NONE', #11224, #5586, #1825 ) ;
#5068=VECTOR ( 'NONE', #9063, 1000.000000000000000 ) ;
#5073=ORIENTED_EDGE ( 'NONE', *, *, #3720, .F. ) ;
#5081=CYLINDRICAL_SURFACE ( 'NONE', #7254, 7.500000000000007105 ) ;
#5088=DIRECTION ( 'NONE',  ( 0.000000000000000000, 0.000000000000000000, 1.000000000000000000 ) ) ;
#5089=ORIENTED_EDGE ( 'NONE', *, *, #3485, .F. ) ;
#5095=UNCERTAINTY_MEASURE_WITH_UNIT (LENGTH_MEASURE( 1.000000000000000082E-05 ), #5744, 'distance_accuracy_value', 'NONE');
#5099=CARTESIAN_POINT ( 'NONE',  ( 45.53315400109643463, 12.00000000000000000, -237.8419396193597208 ) ) ;
#5102=VERTEX_POINT ( 'NONE', #8152 ) ;
#5105=ORIENTED_EDGE ( 'NONE', *, *, #1847, .F. ) ;
#5112=DIRECTION ( 'NONE',  ( -0.000000000000000000, 1.189524669241239115E-16, -1.000000000000000000 ) ) ;
#5120=DIRECTION ( 'NONE',  ( -0.000000000000000000, 1.000000000000000000, 7.930164461608263644E-17 ) ) ;
#5126=CARTESIAN_POINT ( 'NONE',  ( 120.8820948793965186, 12.00000000000000000, -186.6989091883332890 ) ) ;
#5128=DIRECTION ( 'NONE',  ( 0.000000000000000000, 0.000000000000000000, 1.000000000000000000 ) ) ;
#5133=DIRECTION ( 'NONE',  ( -0.000000000000000000, 1.000000000000000000, 7.930164461608263644E-17 ) ) ;
#5135=CARTESIAN_POINT ( 'NONE',  ( 87.04832655144112152, 12.00000000000000000, -217.9289243767383368 ) ) ;
#5146=VERTEX_POINT ( 'NONE', #3498 ) ;
#5154=LINE ( 'NONE', #444, #11398 ) ;
#5158=CYLINDRICAL_SURFACE ( 'NONE', #8168, 7.500000000000007105 ) ;
#5160=VECTOR ( 'NONE', #4561, 1000.000000000000000 ) ;
#5169=EDGE_CURVE ( 'NONE', #10118, #931, #8911, .T. ) ;
#5183=VERTEX_POINT ( 'NONE', #2641 ) ;
#5184=EDGE_CURVE ( 'NONE', #4714, #1702, #6560, .T. ) ;
#5191=VERTEX_POINT ( 'NONE', #3441 ) ;
#5194=AXIS2_PLACEMENT_3D ( 'NONE', #6670, #4012, #7780 ) ;
#5198=CARTESIAN_POINT ( 'NONE',  ( 9.371890508914830252E-13, 152.0000000000000000, -36.42135623730948168 ) ) ;
#5199=ORIENTED_EDGE ( 'NONE', *, *, #3118, .T. ) ;
#5200=ORIENTED_EDGE ( 'NONE', *, *, #3181, .F. ) ;
#5202=CIRCLE ( 'NONE', #12141, 7.500000000000008882 ) ;
#5207=ADVANCED_FACE ( 'NONE', ( #7224 ), #2517, .F. ) ;
#5208=AXIS2_PLACEMENT_3D ( 'NONE', #9113, #2691, #11033 ) ;
#5209=EDGE_LOOP ( 'NONE', ( #11807, #217 ) ) ;
#5214=VERTEX_POINT ( 'NONE', #12045 ) ;
#5215=CARTESIAN_POINT ( 'NONE',  ( 9.371890508914830252E-13, 0.000000000000000000, -36.42135623730949590 ) ) ;
#5223=AXIS2_PLACEMENT_3D ( 'NONE', #838, #6636, #10468 ) ;
#5224=DIRECTION ( 'NONE',  ( -0.000000000000000000, 1.000000000000000000, 7.930164461608263644E-17 ) ) ;
#5227=FACE_BOUND ( 'NONE', #9610, .T. ) ;
#5236=DIRECTION ( 'NONE',  ( 0.000000000000000000, -1.156482317317870246E-16, 1.000000000000000000 ) ) ;
#5242=DIRECTION ( 'NONE',  ( -0.000000000000000000, 1.000000000000000000, -0.000000000000000000 ) ) ;
#5243=DIRECTION ( 'NONE',  ( 0.000000000000000000, -1.000000000000000000, -7.930164461608263644E-17 ) ) ;
#5251=ORIENTED_EDGE ( 'NONE', *, *, #12036, .T. ) ;
#5253=AXIS2_PLACEMENT_3D ( 'NONE', #986, #2900, #1678 ) ;
#5256=EDGE_CURVE ( 'NONE', #1493, #11133, #10212, .T. ) ;
#5257=ORIENTED_EDGE ( 'NONE', *, *, #11914, .F. ) ;
#5263=EDGE_LOOP ( 'NONE', ( #7118, #1286 ) ) ;
#5272=ORIENTED_EDGE ( 'NONE', *, *, #3976, .F. ) ;
#5274=ORIENTED_EDGE ( 'NONE', *, *, #7230, .F. ) ;
#5277=DIRECTION ( 'NONE',  ( 0.000000000000000000, 1.000000000000000000, 0.000000000000000000 ) ) ;
#5278=ORIENTED_EDGE ( 'NONE', *, *, #10098, .F. ) ;
#5283=VECTOR ( 'NONE', #10241, 1000.000000000000000 ) ;
#5284=VECTOR ( 'NONE', #11190, 1000.000000000000000 ) ;
#5287=CARTESIAN_POINT ( 'NONE',  ( 3.123963502971610252E-13, -6.000000000000006217, -88.92135623730948168 ) ) ;
#5293=CARTESIAN_POINT ( 'NONE',  ( 3.123963502971610252E-13, 152.0000000000000000, -96.42135623730948168 ) ) ;
#5294=DIRECTION ( 'NONE',  ( 0.000000000000000000, 0.000000000000000000, -1.000000000000000000 ) ) ;
#5297=FACE_OUTER_BOUND ( 'NONE', #10656, .T. ) ;
#5301=VECTOR ( 'NONE', #3311, 1000.000000000000000 ) ;
#5304=DIRECTION ( 'NONE',  ( -0.000000000000000000, 1.000000000000000000, 0.000000000000000000 ) ) ;
#5310=DIRECTION ( 'NONE',  ( 0.000000000000000000, 0.000000000000000000, 1.000000000000000000 ) ) ;
#5312=CARTESIAN_POINT ( 'NONE',  ( 2.187692937179487324E-12, -6.000000000000004441, 76.07864376269048989 ) ) ;
#5314=DIRECTION ( 'NONE',  ( 0.000000000000000000, 0.000000000000000000, -1.000000000000000000 ) ) ;
#5318=ORIENTED_EDGE ( 'NONE', *, *, #10551, .T. ) ;
#5323=VERTEX_POINT ( 'NONE', #3030 ) ;
#5326=ORIENTED_EDGE ( 'NONE', *, *, #1619, .T. ) ;
#5327=ADVANCED_FACE ( 'NONE', ( #7670 ), #5748, .F. ) ;
#5329=ORIENTED_EDGE ( 'NONE', *, *, #12228, .F. ) ;
#5332=EDGE_CURVE ( 'NONE', #2055, #8525, #3776, .T. ) ;
#5334=DIRECTION ( 'NONE',  ( 0.000000000000000000, 0.000000000000000000, 1.000000000000000000 ) ) ;
#5337=DIRECTION ( 'NONE',  ( 0.000000000000000000, -1.156482317317870246E-16, 1.000000000000000000 ) ) ;
#5338=FACE_OUTER_BOUND ( 'NONE', #6011, .T. ) ;
#5339=DIRECTION ( 'NONE',  ( 0.000000000000000000, 1.000000000000000000, 0.000000000000000000 ) ) ;
#5340=EDGE_LOOP ( 'NONE', ( #7561, #802 ) ) ;
#5345=CARTESIAN_POINT ( 'NONE',  ( 1.561981751485805177E-12, -6.000000000000005329, 23.57864376269050410 ) ) ;
#5351=ORIENTED_EDGE ( 'NONE', *, *, #10852, .F. ) ;
#5355=DIRECTION ( 'NONE',  ( -0.000000000000000000, -1.000000000000000000, -0.000000000000000000 ) ) ;
#5359=VERTEX_POINT ( 'NONE', #10455 ) ;
#5366=CARTESIAN_POINT ( 'NONE',  ( 1.387778780781445676E-14, 0.000000000000000000, 126.4213562373094959 ) ) ;
#5367=DIRECTION ( 'NONE',  ( 0.000000000000000000, 0.000000000000000000, -1.000000000000000000 ) ) ;
#5369=ORIENTED_EDGE ( 'NONE', *, *, #1146, .F. ) ;
#5370=CARTESIAN_POINT ( 'NONE',  ( 6.247927005943220505E-13, 152.0000000000000000, -66.42135623730948168 ) ) ;
#5371=EDGE_CURVE ( 'NONE', #2194, #4285, #8780, .T. ) ;
#5373=DIRECTION ( 'NONE',  ( 0.000000000000000000, 1.000000000000000000, 0.000000000000000000 ) ) ;
#5376=ORIENTED_EDGE ( 'NONE', *, *, #10469, .F. ) ;
#5378=CARTESIAN_POINT ( 'NONE',  ( 1.479627290717497352E-14, -58.00000000000000711, 118.9213562373094817 ) ) ;
#5379=CIRCLE ( 'NONE', #249, 35.00000000000002842 ) ;
#5383=VERTEX_POINT ( 'NONE', #9707 ) ;
#5384=ADVANCED_FACE ( 'NONE', ( #7550, #62, #10511, #4825, #4882, #9464, #1068, #1003, #11379, #3096, #8665, #8721, #8601, #2918, #123, #3898, #177, #3958, #10633, #7727, #11501, #6799, #2111, #5870, #1191, #4944 ), #7794, .F. ) ;
#5385=EDGE_CURVE ( 'NONE', #8245, #7119, #2174, .T. ) ;
#5388=ADVANCED_FACE ( 'NONE', ( #5297 ), #4272, .T. ) ;
#5389=CYLINDRICAL_SURFACE ( 'NONE', #6026, 7.500000000000007105 ) ;
#5390=AXIS2_PLACEMENT_3D ( 'NONE', #11279, #961, #4732 ) ;
#5391=CARTESIAN_POINT ( 'NONE',  ( 35.00000000000000000, 12.00000000000002309, -159.6807709998040252 ) ) ;
#5395=ORIENTED_EDGE ( 'NONE', *, *, #6074, .F. ) ;
#5397=CARTESIAN_POINT ( 'NONE',  ( 3.123963502971610252E-13, 164.0000000000000000, -88.92135623730946747 ) ) ;
#5399=EDGE_LOOP ( 'NONE', ( #7804, #4428 ) ) ;
#5401=DIRECTION ( 'NONE',  ( 0.000000000000000000, 0.000000000000000000, -1.000000000000000000 ) ) ;
#5406=AXIS2_PLACEMENT_3D ( 'NONE', #3463, #10445, #4874 ) ;
#5407=AXIS2_PLACEMENT_3D ( 'NONE', #3981, #4736, #1024 ) ;
#5408=DIRECTION ( 'NONE',  ( -0.000000000000000000, -1.000000000000000000, -0.000000000000000000 ) ) ;
#5416=AXIS2_PLACEMENT_3D ( 'NONE', #4545, #12014, #7257 ) ;
#5417=AXIS2_PLACEMENT_3D ( 'NONE', #2660, #9019, #11132 ) ;
#5419=CARTESIAN_POINT ( 'NONE',  ( 3.123963502971610252E-13, -6.000000000000005329, -96.42135623730949590 ) ) ;
#5432=FACE_OUTER_BOUND ( 'NONE', #10129, .T. ) ;
#5433=ORIENTED_EDGE ( 'NONE', *, *, #7212, .T. ) ;
#5434=DIRECTION ( 'NONE',  ( 0.000000000000000000, 1.000000000000000000, 0.000000000000000000 ) ) ;
#5442=ORIENTED_EDGE ( 'NONE', *, *, #1619, .F. ) ;
#5455=DIRECTION ( 'NONE',  ( 0.000000000000000000, 1.000000000000000000, 0.000000000000000000 ) ) ;
#5456=ADVANCED_FACE ( 'NONE', ( #5994 ), #1539, .F. ) ;
#5464=FACE_OUTER_BOUND ( 'NONE', #9779, .T. ) ;
#5467=ORIENTED_EDGE ( 'NONE', *, *, #4258, .T. ) ;
#5470=AXIS2_PLACEMENT_3D ( 'NONE', #6156, #2441, #5401 ) ;
#5471=LINE ( 'NONE', #5539, #11626 ) ;
#5478=VECTOR ( 'NONE', #4462, 1000.000000000000000 ) ;
#5479=EDGE_CURVE ( 'NONE', #6719, #11656, #8729, .T. ) ;
#5480=EDGE_LOOP ( 'NONE', ( #6150, #675 ) ) ;
#5481=ORIENTED_EDGE ( 'NONE', *, *, #3348, .F. ) ;
#5482=CARTESIAN_POINT ( 'NONE',  ( 0.000000000000000000, 152.0000000000000284, -126.4213562373094959 ) ) ;
#5492=CIRCLE ( 'NONE', #9642, 7.500000000000007105 ) ;
#5496=APPLICATION_CONTEXT ( 'automotive_design' ) ;
#5497=EDGE_CURVE ( 'NONE', #4307, #1330, #11862, .T. ) ;
#5498=AXIS2_PLACEMENT_3D ( 'NONE', #3102, #1490, #9954 ) ;
#5503=CARTESIAN_POINT ( 'NONE',  ( 87.04832655144112152, 12.00000000000000000, -217.9289243767383368 ) ) ;
#5504=CYLINDRICAL_SURFACE ( 'NONE', #7607, 7.500000000000007105 ) ;
#5505=ORIENTED_EDGE ( 'NONE', *, *, #7613, .F. ) ;
#5513=ORIENTED_EDGE ( 'NONE', *, *, #2447, .F. ) ;
#5519=DIRECTION ( 'NONE',  ( 1.000000000000000000, 0.000000000000000000, -0.000000000000000000 ) ) ;
#5520=CIRCLE ( 'NONE', #2766, 7.500000000000007105 ) ;
#5524=FACE_OUTER_BOUND ( 'NONE', #4421, .T. ) ;
#5530=ORIENTED_EDGE ( 'NONE', *, *, #403, .F. ) ;
#5532=EDGE_CURVE ( 'NONE', #11915, #10880, #2212, .T. ) ;
#5539=CARTESIAN_POINT ( 'NONE',  ( 9.371890508914830252E-13, -6.000000000000006217, -28.92135623730948524 ) ) ;
#5544=DIRECTION ( 'NONE',  ( -0.000000000000000000, 1.000000000000000000, 7.930164461608263644E-17 ) ) ;
#5557=VERTEX_POINT ( 'NONE', #543 ) ;
#5565=ORIENTED_EDGE ( 'NONE', *, *, #11914, .T. ) ;
#5566=DIRECTION ( 'NONE',  ( 0.000000000000000000, 1.000000000000000000, 0.000000000000000000 ) ) ;
#5569=VERTEX_POINT ( 'NONE', #4326 ) ;
#5572=ORIENTED_EDGE ( 'NONE', *, *, #9507, .F. ) ;
#5573=AXIS2_PLACEMENT_3D ( 'NONE', #6642, #9484, #4677 ) ;
#5575=AXIS2_PLACEMENT_3D ( 'NONE', #10572, #11441, #9523 ) ;
#5580=EDGE_LOOP ( 'NONE', ( #7078, #3513 ) ) ;
#5582=DIRECTION ( 'NONE',  ( -0.000000000000000000, -1.000000000000000000, -0.000000000000000000 ) ) ;
#5585=CARTESIAN_POINT ( 'NONE',  ( 2.186774452080127126E-12, 152.0000000000000000, 83.57864376269051832 ) ) ;
#5586=DIRECTION ( 'NONE',  ( -0.000000000000000000, 1.000000000000000000, 0.000000000000000000 ) ) ;
#5598=ORIENTED_EDGE ( 'NONE', *, *, #10176, .T. ) ;
#5602=CARTESIAN_POINT ( 'NONE',  ( 35.00000000000000000, 163.9999999999999716, 190.3192290001959748 ) ) ;
#5607=AXIS2_PLACEMENT_3D ( 'NONE', #11543, #10490, #9560 ) ;
#5611=ORIENTED_EDGE ( 'NONE', *, *, #4362, .T. ) ;
#5612=DIRECTION ( 'NONE',  ( 0.000000000000000000, -1.156482317317870246E-16, 1.000000000000000000 ) ) ;
#5613=AXIS2_PLACEMENT_3D ( 'NONE', #10984, #10117, #1585 ) ;
#5614=CIRCLE ( 'NONE', #7596, 7.500000000000013323 ) ;
#5615=VECTOR ( 'NONE', #1216, 1000.000000000000000 ) ;
#5618=EDGE_CURVE ( 'NONE', #1440, #5971, #9714, .T. ) ;
#5619=DIRECTION ( 'NONE',  ( -0.000000000000000000, 1.000000000000000000, -0.000000000000000000 ) ) ;
#5629=CARTESIAN_POINT ( 'NONE',  ( -6.106226635438360972E-13, 12.00000000000000000, -244.6807709998039400 ) ) ;
#5630=CARTESIAN_POINT ( 'NONE',  ( -45.53315400109751465, 12.00000000000000000, -237.8419396193594650 ) ) ;
#5638=ORIENTED_EDGE ( 'NONE', *, *, #8556, .T. ) ;
#5643=EDGE_CURVE ( 'NONE', #7353, #2620, #4198, .T. ) ;
#5650=CARTESIAN_POINT ( 'NONE',  ( 45.53315400109643463, 0.000000000000000000, -237.8419396193597208 ) ) ;
#5656=EDGE_CURVE ( 'NONE', #11947, #10902, #242, .T. ) ;
#5661=ORIENTED_EDGE ( 'NONE', *, *, #11144, .F. ) ;
#5667=CARTESIAN_POINT ( 'NONE',  ( 2.186774452080127126E-12, 163.9999999999999716, 83.57864376269051832 ) ) ;
#5668=VERTEX_POINT ( 'NONE', #9616 ) ;
#5674=DIRECTION ( 'NONE',  ( 0.000000000000000000, 0.000000000000000000, 1.000000000000000000 ) ) ;
#5681=CARTESIAN_POINT ( 'NONE',  ( -144.0488662551579182, 12.00000000000000000, -139.4077238332691877 ) ) ;
#5692=EDGE_LOOP ( 'NONE', ( #6705, #3014 ) ) ;
#5705=ADVANCED_FACE ( 'NONE', ( #11539 ), #4060, .F. ) ;
#5707=AXIS2_PLACEMENT_3D ( 'NONE', #3025, #1985, #9636 ) ;
#5719=ORIENTED_EDGE ( 'NONE', *, *, #4748, .F. ) ;
#5730=ORIENTED_EDGE ( 'NONE', *, *, #3720, .T. ) ;
#5744=( LENGTH_UNIT ( ) NAMED_UNIT ( * ) SI_UNIT ( .MILLI., .METRE. ) );
#5748=CYLINDRICAL_SURFACE ( 'NONE', #5575, 70.00000000000002842 ) ;
#5756=EDGE_CURVE ( 'NONE', #7589, #5668, #11338, .T. ) ;
#5768=EDGE_LOOP ( 'NONE', ( #9987, #7141, #8117, #8990 ) ) ;
#5780=VERTEX_POINT ( 'NONE', #7939 ) ;
#5781=EDGE_CURVE ( 'NONE', #5971, #11527, #8119, .T. ) ;
#5782=CIRCLE ( 'NONE', #7374, 7.500000000000007105 ) ;
#5789=CIRCLE ( 'NONE', #11910, 7.500000000000007105 ) ;
#5795=DIRECTION ( 'NONE',  ( 0.000000000000000000, 0.000000000000000000, 1.000000000000000000 ) ) ;
#5800=CYLINDRICAL_SURFACE ( 'NONE', #5811, 7.500000000000007105 ) ;
#5802=VECTOR ( 'NONE', #5242, 1000.000000000000000 ) ;
#5803=AXIS2_PLACEMENT_3D ( 'NONE', #6555, #115, #6675 ) ;
#5810=CARTESIAN_POINT ( 'NONE',  ( 1.250503886288004501E-12, -6.000000000000004441, -13.92135623730950478 ) ) ;
#5811=AXIS2_PLACEMENT_3D ( 'NONE', #997, #54, #4763 ) ;
#5821=CIRCLE ( 'NONE', #9380, 7.500000000000007105 ) ;
#5835=DIRECTION ( 'NONE',  ( 0.000000000000000000, 1.000000000000000000, 0.000000000000000000 ) ) ;
#5837=ORIENTED_EDGE ( 'NONE', *, *, #2907, .F. ) ;
#5843=VECTOR ( 'NONE', #5887, 1000.000000000000000 ) ;
#5849=VERTEX_POINT ( 'NONE', #7061 ) ;
#5851=CIRCLE ( 'NONE', #4484, 7.500000000000007105 ) ;
#5855=ORIENTED_EDGE ( 'NONE', *, *, #10682, .F. ) ;
#5858=LINE ( 'NONE', #6788, #10441 ) ;
#5868=VECTOR ( 'NONE', #6235, 1000.000000000000000 ) ;
#5870=FACE_BOUND ( 'NONE', #5580, .T. ) ;
#5882=DIRECTION ( 'NONE',  ( 0.000000000000000000, 0.000000000000000000, 1.000000000000000000 ) ) ;
#5885=VECTOR ( 'NONE', #5355, 1000.000000000000000 ) ;
#5887=DIRECTION ( 'NONE',  ( -0.000000000000000000, 1.000000000000000000, 7.930164461608263644E-17 ) ) ;
#5898=ORIENTED_EDGE ( 'NONE', *, *, #5781, .F. ) ;
#5900=VERTEX_POINT ( 'NONE', #384 ) ;
#5901=AXIS2_PLACEMENT_3D ( 'NONE', #56, #10449, #10925 ) ;
#5902=FACE_OUTER_BOUND ( 'NONE', #7513, .T. ) ;
#5912=EDGE_CURVE ( 'NONE', #4307, #10145, #4391, .T. ) ;
#5923=VERTEX_POINT ( 'NONE', #10280 ) ;
#5931=ORIENTED_EDGE ( 'NONE', *, *, #5643, .T. ) ;
#5934=CARTESIAN_POINT ( 'NONE',  ( 1.875296586882326249E-12, 12.00000000000000000, 46.07864376269049700 ) ) ;
#5937=CARTESIAN_POINT ( 'NONE',  ( 1.562900236585165577E-12, -6.000000000000004441, 16.07864376269049700 ) ) ;
#5943=DIRECTION ( 'NONE',  ( -0.000000000000000000, -1.000000000000000000, -0.000000000000000000 ) ) ;
#5944=CYLINDRICAL_SURFACE ( 'NONE', #10344, 7.500000000000007105 ) ;
#5950=FACE_OUTER_BOUND ( 'NONE', #4266, .T. ) ;
#5953=ORIENTED_EDGE ( 'NONE', *, *, #9540, .T. ) ;
#5963=ORIENTED_EDGE ( 'NONE', *, *, #10066, .F. ) ;
#5970=AXIS2_PLACEMENT_3D ( 'NONE', #10220, #1757, #6323 ) ;
#5971=VERTEX_POINT ( 'NONE', #11083 ) ;
#5972=FACE_OUTER_BOUND ( 'NONE', #11294, .T. ) ;
#5982=CIRCLE ( 'NONE', #1642, 7.500000000000007105 ) ;
#5987=ORIENTED_EDGE ( 'NONE', *, *, #3362, .T. ) ;
#5988=DIRECTION ( 'NONE',  ( 0.000000000000000000, 0.000000000000000000, -1.000000000000000000 ) ) ;
#5994=FACE_OUTER_BOUND ( 'NONE', #3138, .T. ) ;
#6003=EDGE_CURVE ( 'NONE', #1493, #10476, #11887, .T. ) ;
#6011=EDGE_LOOP ( 'NONE', ( #8110, #5395, #8180, #5442 ) ) ;
#6019=VERTEX_POINT ( 'NONE', #6383 ) ;
#6026=AXIS2_PLACEMENT_3D ( 'NONE', #9874, #458, #7025 ) ;
#6034=LINE ( 'NONE', #3352, #10084 ) ;
#6037=VERTEX_POINT ( 'NONE', #6449 ) ;
#6039=FACE_OUTER_BOUND ( 'NONE', #10205, .T. ) ;
#6042=LINE ( 'NONE', #9809, #3991 ) ;
#6045=DIRECTION ( 'NONE',  ( 0.000000000000000000, 0.000000000000000000, -1.000000000000000000 ) ) ;
#6046=FACE_BOUND ( 'NONE', #4248, .T. ) ;
#6050=DIRECTION ( 'NONE',  ( -0.000000000000000000, -1.000000000000000000, -0.000000000000000000 ) ) ;
#6055=DIRECTION ( 'NONE',  ( 0.000000000000000000, 0.000000000000000000, 1.000000000000000000 ) ) ;
#6057=VECTOR ( 'NONE', #10080, 1000.000000000000000 ) ;
#6062=EDGE_CURVE ( 'NONE', #11075, #4285, #7756, .T. ) ;
#6064=LINE ( 'NONE', #11868, #8945 ) ;
#6067=ADVANCED_FACE ( 'NONE', ( #12146 ), #11219, .F. ) ;
#6068=CIRCLE ( 'NONE', #5470, 7.500000000000007105 ) ;
#6073=ORIENTED_EDGE ( 'NONE', *, *, #10458, .F. ) ;
#6074=EDGE_CURVE ( 'NONE', #8540, #11819, #8747, .T. ) ;
#6088=DIRECTION ( 'NONE',  ( -0.000000000000000000, -1.000000000000000000, -0.000000000000000000 ) ) ;
#6091=VECTOR ( 'NONE', #790, 1000.000000000000000 ) ;
#6093=CARTESIAN_POINT ( 'NONE',  ( 2.186774452080127126E-12, 0.000000000000000000, 91.07864376269050410 ) ) ;
#6094=AXIS2_PLACEMENT_3D ( 'NONE', #10138, #5434, #8430 ) ;
#6095=ORIENTED_EDGE ( 'NONE', *, *, #8925, .F. ) ;
#6098=ORIENTED_EDGE ( 'NONE', *, *, #2172, .F. ) ;
#6099=DIRECTION ( 'NONE',  ( 0.000000000000000000, 1.000000000000000000, 0.000000000000000000 ) ) ;
#6100=ORIENTED_EDGE ( 'NONE', *, *, #9825, .F. ) ;
#6105=CARTESIAN_POINT ( 'NONE',  ( 1.250503886288004501E-12, 12.00000000000000000, -13.92135623730950300 ) ) ;
#6110=CIRCLE ( 'NONE', #10839, 7.500000000000007105 ) ;
#6112=DIRECTION ( 'NONE',  ( 0.000000000000000000, 1.000000000000000000, 0.000000000000000000 ) ) ;
#6118=FACE_OUTER_BOUND ( 'NONE', #8653, .T. ) ;
#6122=CARTESIAN_POINT ( 'NONE',  ( -151.3258811035894098, 12.00000000000000000, -56.13263083939680342 ) ) ;
#6123=EDGE_LOOP ( 'NONE', ( #1554, #2353 ) ) ;
#6124=FACE_BOUND ( 'NONE', #9309, .T. ) ;
#6142=CARTESIAN_POINT ( 'NONE',  ( -151.3258811035894098, 12.00000000000000000, -56.13263083939680342 ) ) ;
#6146=CIRCLE ( 'NONE', #6339, 70.00000000000002842 ) ;
#6150=ORIENTED_EDGE ( 'NONE', *, *, #2710, .F. ) ;
#6156=CARTESIAN_POINT ( 'NONE',  ( 1.561981751485805177E-12, 163.9999999999999716, 23.57864376269051832 ) ) ;
#6163=CARTESIAN_POINT ( 'NONE',  ( 45.53315400109643463, 0.000000000000000000, -230.3419396193597208 ) ) ;
#6167=DIRECTION ( 'NONE',  ( 0.000000000000000000, 0.000000000000000000, 1.000000000000000000 ) ) ;
#6168=ADVANCED_FACE ( 'NONE', ( #9595 ), #5944, .F. ) ;
#6171=DIRECTION ( 'NONE',  ( 0.000000000000000000, 1.000000000000000000, 0.000000000000000000 ) ) ;
#6172=LINE ( 'NONE', #3088, #2765 ) ;
#6173=VERTEX_POINT ( 'NONE', #3103 ) ;
#6177=EDGE_CURVE ( 'NONE', #4792, #2378, #10465, .T. ) ;
#6179=DIRECTION ( 'NONE',  ( 0.000000000000000000, 0.000000000000000000, 1.000000000000000000 ) ) ;
#6183=FACE_BOUND ( 'NONE', #6961, .T. ) ;
#6185=LINE ( 'NONE', #9951, #2683 ) ;
#6195=CIRCLE ( 'NONE', #5390, 7.500000000000007105 ) ;
#6205=AXIS2_PLACEMENT_3D ( 'NONE', #10248, #2509, #1843 ) ;
#6209=CARTESIAN_POINT ( 'NONE',  ( -35.00000000000000000, 2.428612866367529932E-14, -159.6807709998040252 ) ) ;
#6212=DIRECTION ( 'NONE',  ( 0.000000000000000000, -1.000000000000000000, 0.000000000000000000 ) ) ;
#6215=VERTEX_POINT ( 'NONE', #954 ) ;
#6216=AXIS2_PLACEMENT_3D ( 'NONE', #4392, #9145, #8165 ) ;
#6223=VERTEX_POINT ( 'NONE', #4891 ) ;
#6230=LINE ( 'NONE', #11244, #3337 ) ;
#6232=CARTESIAN_POINT ( 'NONE',  ( 0.000000000000000000, 12.00000000000000000, -89.68077099980401101 ) ) ;
#6235=DIRECTION ( 'NONE',  ( -0.000000000000000000, -1.000000000000000000, -0.000000000000000000 ) ) ;
#6239=FACE_OUTER_BOUND ( 'NONE', #2550, .T. ) ;
#6240=EDGE_CURVE ( 'NONE', #9573, #10609, #4835, .T. ) ;
#6244=AXIS2_PLACEMENT_3D ( 'NONE', #2184, #8734, #5882 ) ;
#6249=DIRECTION ( 'NONE',  ( -0.000000000000000000, -1.000000000000000000, -0.000000000000000000 ) ) ;
#6250=CYLINDRICAL_SURFACE ( 'NONE', #6216, 7.500000000000007105 ) ;
#6252=PRESENTATION_STYLE_ASSIGNMENT (( #11872 ) ) ;
#6253=FACE_OUTER_BOUND ( 'NONE', #9960, .T. ) ;
#6256=CIRCLE ( 'NONE', #3684, 7.500000000000007105 ) ;
#6260=ORIENTED_EDGE ( 'NONE', *, *, #5497, .F. ) ;
#6264=EDGE_LOOP ( 'NONE', ( #8562, #8807 ) ) ;
#6265=EDGE_LOOP ( 'NONE', ( #7537, #10890 ) ) ;
#6274=ORIENTED_EDGE ( 'NONE', *, *, #10993, .F. ) ;
#6275=AXIS2_PLACEMENT_3D ( 'NONE', #4509, #10991, #5236 ) ;
#6287=LINE ( 'NONE', #10055, #2243 ) ;
#6288=CARTESIAN_POINT ( 'NONE',  ( 87.04832655144112152, 0.000000000000000000, -217.9289243767383368 ) ) ;
#6290=VERTEX_POINT ( 'NONE', #1199 ) ;
#6297=ORIENTED_EDGE ( 'NONE', *, *, #11394, .F. ) ;
#6299=CARTESIAN_POINT ( 'NONE',  ( -120.8820948793972434, 12.00000000000000000, -186.6989091883324363 ) ) ;
#6310=CIRCLE ( 'NONE', #9477, 7.500000000000007105 ) ;
#6311=ORIENTED_EDGE ( 'NONE', *, *, #11290, .F. ) ;
#6312=CYLINDRICAL_SURFACE ( 'NONE', #8635, 175.0000000000000284 ) ;
#6315=ORIENTED_EDGE ( 'NONE', *, *, #3995, .T. ) ;
#6316=VERTEX_POINT ( 'NONE', #11698 ) ;
#6320=ORIENTED_EDGE ( 'NONE', *, *, #2370, .T. ) ;
#6321=EDGE_CURVE ( 'NONE', #5183, #8245, #2056, .T. ) ;
#6323=DIRECTION ( 'NONE',  ( 0.000000000000000000, 0.000000000000000000, 1.000000000000000000 ) ) ;
#6324=ORIENTED_EDGE ( 'NONE', *, *, #10471, .F. ) ;
#6339=AXIS2_PLACEMENT_3D ( 'NONE', #6394, #12157, #3600 ) ;
#6343=CIRCLE ( 'NONE', #9510, 35.00000000000000000 ) ;
#6346=CYLINDRICAL_SURFACE ( 'NONE', #11747, 7.500000000000013323 ) ;
#6351=DIRECTION ( 'NONE',  ( 0.000000000000000000, 0.000000000000000000, 1.000000000000000000 ) ) ;
#6357=ORIENTED_EDGE ( 'NONE', *, *, #9540, .F. ) ;
#6362=AXIS2_PLACEMENT_3D ( 'NONE', #3749, #3806, #7401 ) ;
#6365=DIRECTION ( 'NONE',  ( 0.000000000000000000, -1.156482317317870246E-16, 1.000000000000000000 ) ) ;
#6367=CARTESIAN_POINT ( 'NONE',  ( 87.04832655144112152, 12.00000000000000000, -225.4289243767383368 ) ) ;
#6369=EDGE_CURVE ( 'NONE', #2533, #3679, #6064, .T. ) ;
#6371=DIRECTION ( 'NONE',  ( -0.000000000000000000, -1.000000000000000000, -0.000000000000000000 ) ) ;
#6375=ORIENTED_EDGE ( 'NONE', *, *, #3121, .F. ) ;
#6376=EDGE_LOOP ( 'NONE', ( #9486, #4204, #2314, #11824 ) ) ;
#6379=CARTESIAN_POINT ( 'NONE',  ( -6.106226635438360972E-13, 12.00000000000000000, -244.6807709998039400 ) ) ;
#6381=ORIENTED_EDGE ( 'NONE', *, *, #11897, .T. ) ;
#6383=CARTESIAN_POINT ( 'NONE',  ( -35.00000000000000000, 152.0000000000000000, 190.3192290001959748 ) ) ;
#6387=CIRCLE ( 'NONE', #10538, 7.500000000000013323 ) ;
#6389=CYLINDRICAL_SURFACE ( 'NONE', #4692, 7.500000000000007105 ) ;
#6394=CARTESIAN_POINT ( 'NONE',  ( 35.00000000000000000, 81.99999999999998579, 190.3192290001959748 ) ) ;
#6400=DIRECTION ( 'NONE',  ( 0.000000000000000000, 0.000000000000000000, 1.000000000000000000 ) ) ;
#6401=CARTESIAN_POINT ( 'NONE',  ( 1.249585401188644101E-12, 0.000000000000000000, -6.421356237309494119 ) ) ;
#6404=CARTESIAN_POINT ( 'NONE',  ( 0.000000000000000000, 11.99999999999999645, -118.9213562373094817 ) ) ;
#6407=AXIS2_PLACEMENT_3D ( 'NONE', #10657, #3172, #4847 ) ;
#6412=EDGE_LOOP ( 'NONE', ( #9630, #6539, #3370, #6095 ) ) ;
#6414=CARTESIAN_POINT ( 'NONE',  ( -45.53315400109751465, 0.000000000000000000, -237.8419396193594650 ) ) ;
#6418=VECTOR ( 'NONE', #2612, 1000.000000000000000 ) ;
#6419=AXIS2_PLACEMENT_3D ( 'NONE', #1595, #9072, #4325 ) ;
#6421=CARTESIAN_POINT ( 'NONE',  ( 0.000000000000000000, 152.0000000000000284, -118.9213562373094817 ) ) ;
#6428=CARTESIAN_POINT ( 'NONE',  ( 1.387778780781445676E-14, 0.000000000000000000, 126.4213562373094959 ) ) ;
#6431=CARTESIAN_POINT ( 'NONE',  ( 0.000000000000000000, 11.99999999999999645, -126.4213562373094959 ) ) ;
#6438=ORIENTED_EDGE ( 'NONE', *, *, #564, .F. ) ;
#6442=ORIENTED_EDGE ( 'NONE', *, *, #12228, .T. ) ;
#6443=EDGE_CURVE ( 'NONE', #4605, #5780, #3835, .T. ) ;
#6445=DIRECTION ( 'NONE',  ( 0.000000000000000000, 1.000000000000000000, 0.000000000000000000 ) ) ;
#6447=VERTEX_POINT ( 'NONE', #7111 ) ;
#6449=CARTESIAN_POINT ( 'NONE',  ( -35.00000000000000000, 11.99999999999998046, 190.3192290001959748 ) ) ;
#6464=ORIENTED_EDGE ( 'NONE', *, *, #3033, .F. ) ;
#6465=CIRCLE ( 'NONE', #10216, 7.500000000000007105 ) ;
#6466=CARTESIAN_POINT ( 'NONE',  ( 6.247927005943220505E-13, -6.000000000000005329, -66.42135623730949590 ) ) ;
#6469=LINE ( 'NONE', #10110, #6091 ) ;
#6472=CARTESIAN_POINT ( 'NONE',  ( -35.00000000000000000, 152.0000000000000000, -124.6807709998038689 ) ) ;
#6474=CARTESIAN_POINT ( 'NONE',  ( -144.0488662551579182, 12.00000000000000000, -146.9077238332691877 ) ) ;
#6475=VECTOR ( 'NONE', #2297, 1000.000000000000000 ) ;
#6476=EDGE_LOOP ( 'NONE', ( #5274, #3412, #10767, #10154 ) ) ;
#6485=AXIS2_PLACEMENT_3D ( 'NONE', #930, #10370, #5612 ) ;
#6487=EDGE_LOOP ( 'NONE', ( #3353, #3847, #6879, #7407 ) ) ;
#6488=ORIENTED_EDGE ( 'NONE', *, *, #321, .F. ) ;
#6489=FACE_OUTER_BOUND ( 'NONE', #10653, .T. ) ;
#6490=LINE ( 'NONE', #3565, #2864 ) ;
#6492=AXIS2_PLACEMENT_3D ( 'NONE', #3134, #6850, #7962 ) ;
#6505=DIRECTION ( 'NONE',  ( 0.000000000000000000, 0.000000000000000000, 1.000000000000000000 ) ) ;
#6506=DIRECTION ( 'NONE',  ( -1.000000000000000000, -0.000000000000000000, 0.000000000000000000 ) ) ;
#6515=ORIENTED_EDGE ( 'NONE', *, *, #3330, .F. ) ;
#6518=CARTESIAN_POINT ( 'NONE',  ( 151.3258811035896656, 12.00000000000000000, -56.13263083939798292 ) ) ;
#6529=CARTESIAN_POINT ( 'NONE',  ( -126.4213562373094959, 12.00000000000000000, -7.499999999999991118 ) ) ;
#6539=ORIENTED_EDGE ( 'NONE', *, *, #9097, .T. ) ;
#6544=CIRCLE ( 'NONE', #7535, 70.00000000000002842 ) ;
#6545=ORIENTED_EDGE ( 'NONE', *, *, #9288, .F. ) ;
#6548=DIRECTION ( 'NONE',  ( -0.000000000000000000, 1.000000000000000000, 7.930164461608263644E-17 ) ) ;
#6552=ADVANCED_FACE ( 'NONE', ( #1743 ), #11932, .F. ) ;
#6555=CARTESIAN_POINT ( 'NONE',  ( 0.000000000000000000, 11.99999999999999645, -126.4213562373094959 ) ) ;
#6560=CIRCLE ( 'NONE', #9109, 7.500000000000007105 ) ;
#6562=ORIENTED_EDGE ( 'NONE', *, *, #2680, .F. ) ;
#6564=ORIENTED_EDGE ( 'NONE', *, *, #468, .F. ) ;
#6565=EDGE_CURVE ( 'NONE', #8540, #5323, #1670, .T. ) ;
#6577=LINE ( 'NONE', #8385, #3881 ) ;
#6585=FACE_BOUND ( 'NONE', #1750, .T. ) ;
#6595=CIRCLE ( 'NONE', #6205, 7.500000000000007105 ) ;
#6602=ORIENTED_EDGE ( 'NONE', *, *, #8797, .T. ) ;
#6606=EDGE_CURVE ( 'NONE', #7819, #11268, #682, .T. ) ;
#6612=CARTESIAN_POINT ( 'NONE',  ( 1.561981751485805177E-12, -6.000000000000006217, 31.07864376269051121 ) ) ;
#6613=DIRECTION ( 'NONE',  ( 0.000000000000000000, 1.000000000000000000, 0.000000000000000000 ) ) ;
#6615=CIRCLE ( 'NONE', #4650, 7.500000000000013323 ) ;
#6619=EDGE_CURVE ( 'NONE', #647, #8782, #11002, .T. ) ;
#6621=EDGE_LOOP ( 'NONE', ( #4076, #8724 ) ) ;
#6628=DIRECTION ( 'NONE',  ( 0.000000000000000000, 0.000000000000000000, 1.000000000000000000 ) ) ;
#6636=DIRECTION ( 'NONE',  ( 0.000000000000000000, 1.000000000000000000, 0.000000000000000000 ) ) ;
#6639=CYLINDRICAL_SURFACE ( 'NONE', #3403, 7.500000000000007105 ) ;
#6642=CARTESIAN_POINT ( 'NONE',  ( -144.0488662551579182, 0.000000000000000000, -146.9077238332691877 ) ) ;
#6644=ORIENTED_EDGE ( 'NONE', *, *, #1131, .T. ) ;
#6664=CARTESIAN_POINT ( 'NONE',  ( 1.249585401188644101E-12, 152.0000000000000000, -6.421356237309483461 ) ) ;
#6665=EDGE_CURVE ( 'NONE', #4471, #2921, #7585, .T. ) ;
#6666=AXIS2_PLACEMENT_3D ( 'NONE', #134, #9480, #956 ) ;
#6669=VERTEX_POINT ( 'NONE', #5681 ) ;
#6670=CARTESIAN_POINT ( 'NONE',  ( 3.123963502971610252E-13, -6.000000000000005329, -96.42135623730949590 ) ) ;
#6672=FACE_OUTER_BOUND ( 'NONE', #701, .T. ) ;
#6675=DIRECTION ( 'NONE',  ( 0.000000000000000000, 0.000000000000000000, 1.000000000000000000 ) ) ;
#6678=DIRECTION ( 'NONE',  ( -0.000000000000000000, -1.000000000000000000, -0.000000000000000000 ) ) ;
#6687=VERTEX_POINT ( 'NONE', #3770 ) ;
#6692=AXIS2_PLACEMENT_3D ( 'NONE', #3950, #3024, #7601 ) ;
#6693=ORIENTED_EDGE ( 'NONE', *, *, #1319, .T. ) ;
#6695=VECTOR ( 'NONE', #8482, 1000.000000000000000 ) ;
#6698=EDGE_CURVE ( 'NONE', #7241, #64, #6988, .T. ) ;
#6704=LINE ( 'NONE', #9833, #1174 ) ;
#6705=ORIENTED_EDGE ( 'NONE', *, *, #7262, .T. ) ;
#6712=CARTESIAN_POINT ( 'NONE',  ( 0.000000000000000000, 152.0000000000000000, -124.6807709998038689 ) ) ;
#6717=VERTEX_POINT ( 'NONE', #231 ) ;
#6719=VERTEX_POINT ( 'NONE', #7543 ) ;
#6721=DIRECTION ( 'NONE',  ( 0.000000000000000000, 0.000000000000000000, -1.000000000000000000 ) ) ;
#6722=DIRECTION ( 'NONE',  ( -0.000000000000000000, -1.000000000000000000, -0.000000000000000000 ) ) ;
#6726=DIRECTION ( 'NONE',  ( -0.000000000000000000, 1.189524669241239115E-16, -1.000000000000000000 ) ) ;
#6731=( NAMED_UNIT ( * ) PLANE_ANGLE_UNIT ( ) SI_UNIT ( $, .RADIAN. ) );
#6736=CARTESIAN_POINT ( 'NONE',  ( 35.00000000000000000, 0.000000000000000000, 190.3192290001959464 ) ) ;
#6738=EDGE_LOOP ( 'NONE', ( #4756, #8320, #10194, #5505, #832, #852, #1339, #4468, #8355, #10823 ) ) ;
#6739=LINE ( 'NONE', #5810, #482 ) ;
#6740=DIRECTION ( 'NONE',  ( -0.000000000000000000, 1.000000000000000000, 7.930164461608263644E-17 ) ) ;
#6749=VECTOR ( 'NONE', #1614, 1000.000000000000000 ) ;
#6750=VERTEX_POINT ( 'NONE', #8537 ) ;
#6752=DIRECTION ( 'NONE',  ( -0.000000000000000000, -1.000000000000000000, -0.000000000000000000 ) ) ;
#6753=VECTOR ( 'NONE', #4647, 1000.000000000000000 ) ;
#6760=EDGE_LOOP ( 'NONE', ( #3220, #4352 ) ) ;
#6765=EDGE_CURVE ( 'NONE', #4471, #7628, #7606, .T. ) ;
#6766=FACE_OUTER_BOUND ( 'NONE', #9946, .T. ) ;
#6767=CARTESIAN_POINT ( 'NONE',  ( 35.00000000000000000, 81.99999999999998579, 190.3192290001959748 ) ) ;
#6770=EDGE_CURVE ( 'NONE', #7628, #4476, #10353, .T. ) ;
#6782=VECTOR ( 'NONE', #3734, 1000.000000000000000 ) ;
#6784=CARTESIAN_POINT ( 'NONE',  ( 0.000000000000000000, 152.0000000000000000, -124.6807709998038689 ) ) ;
#6788=CARTESIAN_POINT ( 'NONE',  ( 120.8820948793965186, 12.00000000000000000, -194.1989091883332890 ) ) ;
#6792=DIRECTION ( 'NONE',  ( -0.000000000000000000, 1.000000000000000000, 7.930164461608263644E-17 ) ) ;
#6796=CIRCLE ( 'NONE', #11748, 7.500000000000007105 ) ;
#6797=DIRECTION ( 'NONE',  ( 0.000000000000000000, 0.000000000000000000, -1.000000000000000000 ) ) ;
#6799=FACE_BOUND ( 'NONE', #11590, .T. ) ;
#6800=ORIENTED_EDGE ( 'NONE', *, *, #566, .T. ) ;
#6806=DIRECTION ( 'NONE',  ( 1.000000000000000000, 0.000000000000000000, -0.000000000000000000 ) ) ;
#6815=CIRCLE ( 'NONE', #10960, 7.500000000000007105 ) ;
#6816=EDGE_LOOP ( 'NONE', ( #7795, #11766 ) ) ;
#6819=LINE ( 'NONE', #2992, #720 ) ;
#6826=( GEOMETRIC_REPRESENTATION_CONTEXT ( 3 ) GLOBAL_UNCERTAINTY_ASSIGNED_CONTEXT ( ( #5095 ) ) GLOBAL_UNIT_ASSIGNED_CONTEXT ( ( #5744, #6731, #7487 ) ) REPRESENTATION_CONTEXT ( 'NONE', 'WORKASPACE' ) );
#6828=CARTESIAN_POINT ( 'NONE',  ( 3.123963502971610252E-13, 0.000000000000000000, -96.42135623730949590 ) ) ;
#6836=VECTOR ( 'NONE', #11460, 1000.000000000000000 ) ;
#6841=CARTESIAN_POINT ( 'NONE',  ( 144.0488662551573782, 12.00000000000000000, -146.9077238332702109 ) ) ;
#6847=CIRCLE ( 'NONE', #1508, 7.500000000000007105 ) ;
#6850=DIRECTION ( 'NONE',  ( -0.000000000000000000, -1.000000000000000000, -0.000000000000000000 ) ) ;
#6853=EDGE_CURVE ( 'NONE', #4605, #8531, #9459, .T. ) ;
#6855=EDGE_CURVE ( 'NONE', #6223, #9369, #6997, .T. ) ;
#6864=DIRECTION ( 'NONE',  ( 0.000000000000000000, 1.000000000000000000, 0.000000000000000000 ) ) ;
#6869=ORIENTED_EDGE ( 'NONE', *, *, #11620, .F. ) ;
#6874=CARTESIAN_POINT ( 'NONE',  ( -126.4213562373094959, 12.00000000000000000, 7.500000000000036415 ) ) ;
#6875=DIRECTION ( 'NONE',  ( -0.000000000000000000, 1.000000000000000000, 7.930164461608263644E-17 ) ) ;
#6879=ORIENTED_EDGE ( 'NONE', *, *, #1844, .T. ) ;
#6886=ORIENTED_EDGE ( 'NONE', *, *, #11356, .F. ) ;
#6888=CYLINDRICAL_SURFACE ( 'NONE', #8585, 7.500000000000007105 ) ;
#6890=PRODUCT_CONTEXT ( 'NONE', #5496, 'mechanical' ) ;
#6893=DIRECTION ( 'NONE',  ( -1.000000000000000000, -0.000000000000000000, -0.000000000000000000 ) ) ;
#6901=EDGE_CURVE ( 'NONE', #1936, #10559, #3427, .T. ) ;
#6909=ORIENTED_EDGE ( 'NONE', *, *, #2840, .T. ) ;
#6913=DIRECTION ( 'NONE',  ( 0.000000000000000000, 0.000000000000000000, -1.000000000000000000 ) ) ;
#6920=DIRECTION ( 'NONE',  ( 0.000000000000000000, 1.000000000000000000, 0.000000000000000000 ) ) ;
#6926=ORIENTED_EDGE ( 'NONE', *, *, #9644, .F. ) ;
#6939=AXIS2_PLACEMENT_3D ( 'NONE', #10539, #208, #3993 ) ;
#6946=ORIENTED_EDGE ( 'NONE', *, *, #11769, .T. ) ;
#6947=DIRECTION ( 'NONE',  ( 0.000000000000000000, 1.000000000000000000, 0.000000000000000000 ) ) ;
#6955=UNCERTAINTY_MEASURE_WITH_UNIT (LENGTH_MEASURE( 1.000000000000000082E-05 ), #1676, 'distance_accuracy_value', 'NONE');
#6961=EDGE_LOOP ( 'NONE', ( #189, #10780 ) ) ;
#6966=CARTESIAN_POINT ( 'NONE',  ( 3.133148353965215262E-13, 12.00000000000000000, -103.9213562373094959 ) ) ;
#6967=EDGE_CURVE ( 'NONE', #1856, #3561, #8185, .T. ) ;
#6971=FACE_BOUND ( 'NONE', #11257, .T. ) ;
#6975=ORIENTED_EDGE ( 'NONE', *, *, #4276, .T. ) ;
#6978=ADVANCED_FACE ( 'NONE', ( #2561 ), #8132, .F. ) ;
#6979=CARTESIAN_POINT ( 'NONE',  ( 1.561981751485805177E-12, -6.000000000000005329, 23.57864376269050410 ) ) ;
#6982=DIRECTION ( 'NONE',  ( -0.000000000000000000, 1.000000000000000000, 7.930164461608263644E-17 ) ) ;
#6986=CIRCLE ( 'NONE', #1273, 7.500000000000008882 ) ;
#6988=CIRCLE ( 'NONE', #9571, 175.0000000000000000 ) ;
#6991=CARTESIAN_POINT ( 'NONE',  ( -151.3258811035894098, 0.000000000000000000, -56.13263083939680342 ) ) ;
#6994=ORIENTED_EDGE ( 'NONE', *, *, #4752, .T. ) ;
#6997=CIRCLE ( 'NONE', #5406, 7.500000000000007105 ) ;
#7001=EDGE_LOOP ( 'NONE', ( #5073, #10412 ) ) ;
#7003=CARTESIAN_POINT ( 'NONE',  ( -154.5043356068770493, 0.000000000000000000, -94.56666130601601594 ) ) ;
#7007=AXIS2_PLACEMENT_3D ( 'NONE', #10223, #10160, #3469 ) ;
#7008=ORIENTED_EDGE ( 'NONE', *, *, #3828, .F. ) ;
#7025=DIRECTION ( 'NONE',  ( 0.000000000000000000, 0.000000000000000000, -1.000000000000000000 ) ) ;
#7031=FACE_BOUND ( 'NONE', #3840, .T. ) ;
#7032=CYLINDRICAL_SURFACE ( 'NONE', #3730, 7.500000000000007105 ) ;
#7042=VERTEX_POINT ( 'NONE', #5397 ) ;
#7043=ORIENTED_EDGE ( 'NONE', *, *, #3501, .T. ) ;
#7047=AXIS2_PLACEMENT_3D ( 'NONE', #5630, #5566, #4656 ) ;
#7048=DIRECTION ( 'NONE',  ( -0.000000000000000000, 1.000000000000000000, 7.930164461608263644E-17 ) ) ;
#7050=DIRECTION ( 'NONE',  ( -0.000000000000000000, -1.000000000000000000, -0.000000000000000000 ) ) ;
#7053=ADVANCED_FACE ( 'NONE', ( #11165, #10352, #6585, #4554, #12218, #1895, #7570, #3741, #3538, #10236 ), #8265, .F. ) ;
#7056=ORIENTED_EDGE ( 'NONE', *, *, #5656, .F. ) ;
#7061=CARTESIAN_POINT ( 'NONE',  ( 1.562900236585165577E-12, 0.000000000000000000, 16.07864376269049700 ) ) ;
#7063=CIRCLE ( 'NONE', #3915, 7.500000000000007105 ) ;
#7065=ORIENTED_EDGE ( 'NONE', *, *, #6240, .F. ) ;
#7067=LINE ( 'NONE', #1506, #9963 ) ;
#7073=VECTOR ( 'NONE', #4927, 1000.000000000000000 ) ;
#7074=ADVANCED_FACE ( 'NONE', ( #5464 ), #8459, .F. ) ;
#7075=ORIENTED_EDGE ( 'NONE', *, *, #2976, .T. ) ;
#7078=ORIENTED_EDGE ( 'NONE', *, *, #11470, .T. ) ;
#7081=CARTESIAN_POINT ( 'NONE',  ( 0.000000000000000000, -58.00000000000000711, -126.4213562373094959 ) ) ;
#7084=CARTESIAN_POINT ( 'NONE',  ( -45.53315400109751465, 12.00000000000000000, -237.8419396193594650 ) ) ;
#7088=FACE_OUTER_BOUND ( 'NONE', #8787, .T. ) ;
#7090=DIRECTION ( 'NONE',  ( 0.000000000000000000, 1.000000000000000000, 0.000000000000000000 ) ) ;
#7092=CIRCLE ( 'NONE', #1777, 7.500000000000007105 ) ;
#7098=EDGE_LOOP ( 'NONE', ( #1793, #9612, #2176, #2956, #11314 ) ) ;
#7111=CARTESIAN_POINT ( 'NONE',  ( -45.53315400109751465, 0.000000000000000000, -230.3419396193594366 ) ) ;
#7113=FACE_OUTER_BOUND ( 'NONE', #11007, .T. ) ;
#7115=CARTESIAN_POINT ( 'NONE',  ( 120.8820948793965186, 12.00000000000000000, -186.6989091883332890 ) ) ;
#7118=ORIENTED_EDGE ( 'NONE', *, *, #3820, .T. ) ;
#7119=VERTEX_POINT ( 'NONE', #11530 ) ;
#7120=ADVANCED_FACE ( 'NONE', ( #5902 ), #6888, .F. ) ;
#7121=CARTESIAN_POINT ( 'NONE',  ( 1.250503886288004501E-12, 152.0000000000000000, -13.92135623730949234 ) ) ;
#7123=EDGE_CURVE ( 'NONE', #1455, #9404, #5614, .T. ) ;
#7126=ORIENTED_EDGE ( 'NONE', *, *, #2976, .F. ) ;
#7128=ORIENTED_EDGE ( 'NONE', *, *, #3655, .T. ) ;
#7137=ORIENTED_EDGE ( 'NONE', *, *, #4752, .F. ) ;
#7138=FACE_OUTER_BOUND ( 'NONE', #328, .T. ) ;
#7141=ORIENTED_EDGE ( 'NONE', *, *, #7686, .T. ) ;
#7145=ORIENTED_EDGE ( 'NONE', *, *, #9458, .F. ) ;
#7149=PRODUCT_DEFINITION ( 'UNKNOWN', '', #9202, #3808 ) ;
#7155=FACE_BOUND ( 'NONE', #11565, .T. ) ;
#7156=CARTESIAN_POINT ( 'NONE',  ( 144.0488662551573782, 0.000000000000000000, -146.9077238332702109 ) ) ;
#7159=ADVANCED_FACE ( 'NONE', ( #9066 ), #6346, .F. ) ;
#7167=EDGE_LOOP ( 'NONE', ( #10598, #10146 ) ) ;
#7175=CARTESIAN_POINT ( 'NONE',  ( 1.387778780781445676E-14, -58.00000000000000711, 126.4213562373094959 ) ) ;
#7176=CYLINDRICAL_SURFACE ( 'NONE', #11243, 7.500000000000007105 ) ;
#7181=VERTEX_POINT ( 'NONE', #1724 ) ;
#7184=AXIS2_PLACEMENT_3D ( 'NONE', #7486, #11067, #2592 ) ;
#7193=AXIS2_PLACEMENT_3D ( 'NONE', #2738, #6506, #2116 ) ;
#7196=CARTESIAN_POINT ( 'NONE',  ( 2.186774452080127126E-12, -6.000000000000005329, 83.57864376269050410 ) ) ;
#7206=CARTESIAN_POINT ( 'NONE',  ( 1.561981751485805177E-12, 12.00000000000000000, 31.07864376269051121 ) ) ;
#7212=EDGE_CURVE ( 'NONE', #2514, #11133, #5202, .T. ) ;
#7215=DIRECTION ( 'NONE',  ( -1.000000000000000000, -0.000000000000000000, -0.000000000000000000 ) ) ;
#7217=DIRECTION ( 'NONE',  ( 0.000000000000000000, 0.000000000000000000, -1.000000000000000000 ) ) ;
#7218=CARTESIAN_POINT ( 'NONE',  ( -144.0488662551579182, 12.00000000000000000, -146.9077238332691877 ) ) ;
#7221=VERTEX_POINT ( 'NONE', #2999 ) ;
#7224=FACE_OUTER_BOUND ( 'NONE', #10021, .T. ) ;
#7226=CARTESIAN_POINT ( 'NONE',  ( 1.387778780781445676E-14, -58.00000000000000711, 133.9213562373095101 ) ) ;
#7228=EDGE_CURVE ( 'NONE', #2921, #4471, #4828, .T. ) ;
#7230=EDGE_CURVE ( 'NONE', #8717, #8333, #10362, .T. ) ;
#7231=VERTEX_POINT ( 'NONE', #2077 ) ;
#7232=CIRCLE ( 'NONE', #1504, 7.500000000000007105 ) ;
#7241=VERTEX_POINT ( 'NONE', #4967 ) ;
#7246=ORIENTED_EDGE ( 'NONE', *, *, #3053, .F. ) ;
#7254=AXIS2_PLACEMENT_3D ( 'NONE', #6299, #8856, #4387 ) ;
#7256=EDGE_LOOP ( 'NONE', ( #9084, #11649, #11607, #7853 ) ) ;
#7257=DIRECTION ( 'NONE',  ( 0.000000000000000000, 0.000000000000000000, 1.000000000000000000 ) ) ;
#7258=DIRECTION ( 'NONE',  ( 0.000000000000000000, 0.000000000000000000, 1.000000000000000000 ) ) ;
#7259=DIRECTION ( 'NONE',  ( -0.000000000000000000, -1.000000000000000000, -0.000000000000000000 ) ) ;
#7260=DIRECTION ( 'NONE',  ( 0.000000000000000000, 0.000000000000000000, 1.000000000000000000 ) ) ;
#7262=EDGE_CURVE ( 'NONE', #4792, #3812, #474, .T. ) ;
#7267=CARTESIAN_POINT ( 'NONE',  ( 35.00000000000000000, 81.99999999999998579, -124.6807709998039826 ) ) ;
#7275=DIRECTION ( 'NONE',  ( 0.000000000000000000, -1.156482317317870246E-16, 1.000000000000000000 ) ) ;
#7277=DIRECTION ( 'NONE',  ( 0.000000000000000000, -1.000000000000000000, -7.930164461608263644E-17 ) ) ;
#7279=ORIENTED_EDGE ( 'NONE', *, *, #10327, .F. ) ;
#7280=DIRECTION ( 'NONE',  ( 0.000000000000000000, 1.000000000000000000, 0.000000000000000000 ) ) ;
#7283=AXIS2_PLACEMENT_3D ( 'NONE', #12053, #6613, #2784 ) ;
#7287=CARTESIAN_POINT ( 'NONE',  ( 0.000000000000000000, -58.00000000000000711, -126.4213562373094959 ) ) ;
#7288=DIRECTION ( 'NONE',  ( 0.000000000000000000, 0.000000000000000000, -1.000000000000000000 ) ) ;
#7290=EDGE_CURVE ( 'NONE', #2055, #4489, #5821, .T. ) ;
#7293=CIRCLE ( 'NONE', #4328, 7.500000000000007105 ) ;
#7298=DIRECTION ( 'NONE',  ( 0.000000000000000000, 1.000000000000000000, 0.000000000000000000 ) ) ;
#7301=DIRECTION ( 'NONE',  ( 0.000000000000000000, 1.000000000000000000, 0.000000000000000000 ) ) ;
#7304=PLANE ( 'NONE',  #4241 ) ;
#7310=CARTESIAN_POINT ( 'NONE',  ( 9.371890508914830252E-13, 152.0000000000000000, -28.92135623730947458 ) ) ;
#7313=ADVANCED_FACE ( 'NONE', ( #1864 ), #3514, .F. ) ;
#7320=ADVANCED_FACE ( 'NONE', ( #9461 ), #819, .F. ) ;
#7324=CARTESIAN_POINT ( 'NONE',  ( 3.123963502971610252E-13, 0.000000000000000000, -96.42135623730949590 ) ) ;
#7334=CARTESIAN_POINT ( 'NONE',  ( 144.0488662551573782, 12.00000000000000000, -139.4077238332702109 ) ) ;
#7336=LINE ( 'NONE', #6472, #10057 ) ;
#7344=EDGE_LOOP ( 'NONE', ( #1980, #2708, #984, #1096 ) ) ;
#7352=EDGE_CURVE ( 'NONE', #10844, #4515, #10952, .T. ) ;
#7353=VERTEX_POINT ( 'NONE', #12096 ) ;
#7356=CARTESIAN_POINT ( 'NONE',  ( 35.00000000000000000, 81.99999999999998579, 272.3192290001959464 ) ) ;
#7359=EDGE_CURVE ( 'NONE', #4907, #7819, #3481, .T. ) ;
#7364=DIRECTION ( 'NONE',  ( 0.000000000000000000, 0.000000000000000000, 1.000000000000000000 ) ) ;
#7366=EDGE_LOOP ( 'NONE', ( #6545, #6320, #10956, #55 ) ) ;
#7369=ORIENTED_EDGE ( 'NONE', *, *, #1201, .T. ) ;
#7371=EDGE_CURVE ( 'NONE', #2076, #4751, #287, .T. ) ;
#7374=AXIS2_PLACEMENT_3D ( 'NONE', #6414, #799, #10056 ) ;
#7382=AXIS2_PLACEMENT_3D ( 'NONE', #4757, #8532, #1234 ) ;
#7388=DIRECTION ( 'NONE',  ( 0.000000000000000000, 0.000000000000000000, 1.000000000000000000 ) ) ;
#7391=CIRCLE ( 'NONE', #891, 7.500000000000007105 ) ;
#7396=ORIENTED_EDGE ( 'NONE', *, *, #5479, .T. ) ;
#7401=DIRECTION ( 'NONE',  ( 0.000000000000000000, 0.000000000000000000, 1.000000000000000000 ) ) ;
#7402=AXIS2_PLACEMENT_3D ( 'NONE', #881, #4654, #2913 ) ;
#7406=ORIENTED_EDGE ( 'NONE', *, *, #6901, .T. ) ;
#7407=ORIENTED_EDGE ( 'NONE', *, *, #7508, .F. ) ;
#7409=ORIENTED_EDGE ( 'NONE', *, *, #6770, .T. ) ;
#7416=ORIENTED_EDGE ( 'NONE', *, *, #9158, .F. ) ;
#7437=CARTESIAN_POINT ( 'NONE',  ( 9.371890508914830252E-13, -6.000000000000005329, -36.42135623730949590 ) ) ;
#7441=CARTESIAN_POINT ( 'NONE',  ( 9.184850993605159777E-16, -58.00000000000000711, -133.9213562373095101 ) ) ;
#7451=EDGE_CURVE ( 'NONE', #12119, #4907, #11352, .T. ) ;
#7454=EDGE_CURVE ( 'NONE', #10844, #1640, #6739, .T. ) ;
#7456=AXIS2_PLACEMENT_3D ( 'NONE', #1621, #763, #10955 ) ;
#7459=DIRECTION ( 'NONE',  ( 0.000000000000000000, 1.000000000000000000, 0.000000000000000000 ) ) ;
#7463=EDGE_CURVE ( 'NONE', #3418, #3398, #4053, .T. ) ;
#7477=ORIENTED_EDGE ( 'NONE', *, *, #4033, .F. ) ;
#7486=CARTESIAN_POINT ( 'NONE',  ( 0.000000000000000000, 0.000000000000000000, -126.4213562373094959 ) ) ;
#7487=( NAMED_UNIT ( * ) SI_UNIT ( $, .STERADIAN. ) SOLID_ANGLE_UNIT ( ) );
#7489=LINE ( 'NONE', #1675, #12227 ) ;
#7495=ORIENTED_EDGE ( 'NONE', *, *, #6003, .F. ) ;
#7503=DIRECTION ( 'NONE',  ( 0.000000000000000000, -1.156482317317870246E-16, 1.000000000000000000 ) ) ;
#7504=VERTEX_POINT ( 'NONE', #2922 ) ;
#7505=EDGE_CURVE ( 'NONE', #5900, #9223, #1072, .T. ) ;
#7506=DIRECTION ( 'NONE',  ( 0.000000000000000000, 0.000000000000000000, -1.000000000000000000 ) ) ;
#7507=LINE ( 'NONE', #841, #4024 ) ;
#7508=EDGE_CURVE ( 'NONE', #2620, #7353, #6615, .T. ) ;
#7511=DIRECTION ( 'NONE',  ( -0.000000000000000000, 1.000000000000000000, 0.000000000000000000 ) ) ;
#7513=EDGE_LOOP ( 'NONE', ( #5719, #1903, #4682, #889 ) ) ;
#7517=DIRECTION ( 'NONE',  ( -0.000000000000000000, 1.000000000000000000, 7.930164461608263644E-17 ) ) ;
#7520=DIRECTION ( 'NONE',  ( 0.000000000000000000, 0.000000000000000000, 1.000000000000000000 ) ) ;
#7524=DIRECTION ( 'NONE',  ( 0.000000000000000000, 1.000000000000000000, 0.000000000000000000 ) ) ;
#7528=CYLINDRICAL_SURFACE ( 'NONE', #7769, 7.500000000000007105 ) ;
#7530=ORIENTED_EDGE ( 'NONE', *, *, #11971, .T. ) ;
#7534=CARTESIAN_POINT ( 'NONE',  ( 0.000000000000000000, 12.00000000000000000, -89.68077099980401101 ) ) ;
#7535=AXIS2_PLACEMENT_3D ( 'NONE', #3309, #2158, #10614 ) ;
#7537=ORIENTED_EDGE ( 'NONE', *, *, #7123, .F. ) ;
#7543=CARTESIAN_POINT ( 'NONE',  ( -87.04832655144203102, 12.00000000000000000, -210.4289243767376831 ) ) ;
#7545=ORIENTED_EDGE ( 'NONE', *, *, #5371, .F. ) ;
#7546=VECTOR ( 'NONE', #9823, 1000.000000000000000 ) ;
#7550=FACE_BOUND ( 'NONE', #2436, .T. ) ;
#7552=ORIENTED_EDGE ( 'NONE', *, *, #9499, .T. ) ;
#7553=AXIS2_PLACEMENT_3D ( 'NONE', #7826, #11600, #3871 ) ;
#7554=DIRECTION ( 'NONE',  ( -0.000000000000000000, -1.000000000000000000, -0.000000000000000000 ) ) ;
#7556=ORIENTED_EDGE ( 'NONE', *, *, #4675, .T. ) ;
#7561=ORIENTED_EDGE ( 'NONE', *, *, #10615, .F. ) ;
#7563=CARTESIAN_POINT ( 'NONE',  ( -6.106226635438360972E-13, 0.000000000000000000, -244.6807709998039400 ) ) ;
#7570=FACE_BOUND ( 'NONE', #6816, .T. ) ;
#7577=EDGE_CURVE ( 'NONE', #8293, #8781, #8198, .T. ) ;
#7579=DIRECTION ( 'NONE',  ( 0.000000000000000000, 1.000000000000000000, 2.312964634635740689E-15 ) ) ;
#7580=DIRECTION ( 'NONE',  ( 0.000000000000000000, 0.000000000000000000, 1.000000000000000000 ) ) ;
#7584=AXIS2_PLACEMENT_3D ( 'NONE', #6474, #796, #8280 ) ;
#7585=CIRCLE ( 'NONE', #7184, 7.500000000000007105 ) ;
#7589=VERTEX_POINT ( 'NONE', #9359 ) ;
#7592=FACE_OUTER_BOUND ( 'NONE', #11236, .T. ) ;
#7594=DIRECTION ( 'NONE',  ( 0.000000000000000000, 1.000000000000000000, 0.000000000000000000 ) ) ;
#7596=AXIS2_PLACEMENT_3D ( 'NONE', #4541, #11149, #1919 ) ;
#7598=ORIENTED_EDGE ( 'NONE', *, *, #9981, .F. ) ;
#7599=DIRECTION ( 'NONE',  ( 0.000000000000000000, 1.000000000000000000, 0.000000000000000000 ) ) ;
#7601=DIRECTION ( 'NONE',  ( 0.000000000000000000, 0.000000000000000000, -1.000000000000000000 ) ) ;
#7604=AXIS2_PLACEMENT_3D ( 'NONE', #8387, #1404, #2679 ) ;
#7606=LINE ( 'NONE', #2787, #3047 ) ;
#7607=AXIS2_PLACEMENT_3D ( 'NONE', #7175, #1548, #5310 ) ;
#7609=ORIENTED_EDGE ( 'NONE', *, *, #2581, .F. ) ;
#7610=DIRECTION ( 'NONE',  ( -0.000000000000000000, 1.000000000000000000, 7.930164461608263644E-17 ) ) ;
#7612=ADVANCED_FACE ( 'NONE', ( #11731 ), #5389, .F. ) ;
#7613=EDGE_CURVE ( 'NONE', #5102, #6019, #693, .T. ) ;
#7614=DIRECTION ( 'NONE',  ( -1.000000000000000000, -0.000000000000000000, -0.000000000000000000 ) ) ;
#7628=VERTEX_POINT ( 'NONE', #3594 ) ;
#7636=ORIENTED_EDGE ( 'NONE', *, *, #5256, .F. ) ;
#7641=CARTESIAN_POINT ( 'NONE',  ( 1.479627290717497352E-14, 163.9999999999999716, 118.9213562373094817 ) ) ;
#7645=DIRECTION ( 'NONE',  ( 0.000000000000000000, 0.000000000000000000, 1.000000000000000000 ) ) ;
#7647=ORIENTED_EDGE ( 'NONE', *, *, #1558, .F. ) ;
#7654=DIRECTION ( 'NONE',  ( -0.000000000000000000, 1.000000000000000000, 0.000000000000000000 ) ) ;
#7659=ADVANCED_FACE ( 'NONE', ( #9169 ), #8187, .F. ) ;
#7661=DIRECTION ( 'NONE',  ( 0.000000000000000000, 1.000000000000000000, 0.000000000000000000 ) ) ;
#7667=EDGE_CURVE ( 'NONE', #502, #2477, #11753, .T. ) ;
#7670=FACE_OUTER_BOUND ( 'NONE', #9347, .T. ) ;
#7672=AXIS2_PLACEMENT_3D ( 'NONE', #8926, #455, #8664 ) ;
#7673=EDGE_LOOP ( 'NONE', ( #1, #5565, #4224, #797 ) ) ;
#7675=DIRECTION ( 'NONE',  ( -0.000000000000000000, 1.000000000000000000, 7.930164461608263644E-17 ) ) ;
#7686=EDGE_CURVE ( 'NONE', #125, #739, #12083, .T. ) ;
#7698=DIRECTION ( 'NONE',  ( 0.000000000000000000, -1.156482317317870246E-16, 1.000000000000000000 ) ) ;
#7711=DIRECTION ( 'NONE',  ( 0.000000000000000000, 1.000000000000000000, 0.000000000000000000 ) ) ;
#7716=CARTESIAN_POINT ( 'NONE',  ( 87.04832655144112152, 0.000000000000000000, -217.9289243767383368 ) ) ;
#7719=AXIS2_PLACEMENT_3D ( 'NONE', #5099, #8916, #4122 ) ;
#7723=EDGE_CURVE ( 'NONE', #8695, #3054, #3652, .T. ) ;
#7727=FACE_BOUND ( 'NONE', #4399, .T. ) ;
#7729=ORIENTED_EDGE ( 'NONE', *, *, #6443, .T. ) ;
#7733=PLANE ( 'NONE',  #7193 ) ;
#7740=CARTESIAN_POINT ( 'NONE',  ( 35.00000000000000000, -4.436643353671145300E-15, 81.78351099501843180 ) ) ;
#7750=CARTESIAN_POINT ( 'NONE',  ( 3.123963502971610252E-13, 152.0000000000000000, -96.42135623730948168 ) ) ;
#7754=CARTESIAN_POINT ( 'NONE',  ( 35.00000000000000000, 152.0000000000000000, 190.3192290001959748 ) ) ;
#7756=CIRCLE ( 'NONE', #3796, 81.99999999999998579 ) ;
#7757=ORIENTED_EDGE ( 'NONE', *, *, #4748, .T. ) ;
#7762=FACE_OUTER_BOUND ( 'NONE', #897, .T. ) ;
#7769=AXIS2_PLACEMENT_3D ( 'NONE', #2512, #2706, #1587 ) ;
#7773=ORIENTED_EDGE ( 'NONE', *, *, #733, .F. ) ;
#7775=CARTESIAN_POINT ( 'NONE',  ( 1.874378101782966050E-12, -6.000000000000005329, 53.57864376269050410 ) ) ;
#7779=ORIENTED_EDGE ( 'NONE', *, *, #3264, .F. ) ;
#7780=DIRECTION ( 'NONE',  ( 0.000000000000000000, -1.156482317317870246E-16, 1.000000000000000000 ) ) ;
#7782=CARTESIAN_POINT ( 'NONE',  ( 0.000000000000000000, 0.000000000000000000, -224.6807709998039968 ) ) ;
#7787=CIRCLE ( 'NONE', #4422, 7.500000000000007105 ) ;
#7789=AXIS2_PLACEMENT_3D ( 'NONE', #9241, #12093, #7698 ) ;
#7793=DIRECTION ( 'NONE',  ( 0.000000000000000000, 0.000000000000000000, 1.000000000000000000 ) ) ;
#7794=PLANE ( 'NONE',  #3192 ) ;
#7795=ORIENTED_EDGE ( 'NONE', *, *, #2615, .T. ) ;
#7800=CIRCLE ( 'NONE', #11554, 7.500000000000020428 ) ;
#7804=ORIENTED_EDGE ( 'NONE', *, *, #9627, .T. ) ;
#7812=CYLINDRICAL_SURFACE ( 'NONE', #10388, 175.0000000000000284 ) ;
#7814=CYLINDRICAL_SURFACE ( 'NONE', #9268, 7.500000000000020428 ) ;
#7817=AXIS2_PLACEMENT_3D ( 'NONE', #11574, #7866, #9771 ) ;
#7819=VERTEX_POINT ( 'NONE', #11454 ) ;
#7821=EDGE_LOOP ( 'NONE', ( #4506, #3975, #11396, #10570 ) ) ;
#7823=ORIENTED_EDGE ( 'NONE', *, *, #2018, .F. ) ;
#7826=CARTESIAN_POINT ( 'NONE',  ( 1.561981751485805177E-12, -6.000000000000005329, 23.57864376269050410 ) ) ;
#7829=CARTESIAN_POINT ( 'NONE',  ( 9.381075359908434252E-13, 0.000000000000000000, -43.92135623730950300 ) ) ;
#7833=DIRECTION ( 'NONE',  ( -0.000000000000000000, 1.000000000000000000, 7.930164461608263644E-17 ) ) ;
#7835=ORIENTED_EDGE ( 'NONE', *, *, #7686, .F. ) ;
#7837=AXIS2_PLACEMENT_3D ( 'NONE', #7196, #10965, #333 ) ;
#7838=ORIENTED_EDGE ( 'NONE', *, *, #2710, .T. ) ;
#7845=ORIENTED_EDGE ( 'NONE', *, *, #2583, .F. ) ;
#7848=DIRECTION ( 'NONE',  ( -0.000000000000000000, -1.000000000000000000, -0.000000000000000000 ) ) ;
#7853=ORIENTED_EDGE ( 'NONE', *, *, #3828, .T. ) ;
#7854=DIRECTION ( 'NONE',  ( 0.000000000000000000, 0.000000000000000000, 1.000000000000000000 ) ) ;
#7856=DIRECTION ( 'NONE',  ( 0.000000000000000000, 0.000000000000000000, -1.000000000000000000 ) ) ;
#7866=DIRECTION ( 'NONE',  ( -0.000000000000000000, -1.000000000000000000, -0.000000000000000000 ) ) ;
#7867=VECTOR ( 'NONE', #8153, 1000.000000000000000 ) ;
#7874=CIRCLE ( 'NONE', #5901, 7.500000000000007105 ) ;
#7882=CARTESIAN_POINT ( 'NONE',  ( -154.5043356068770493, 12.00000000000000000, -109.5666613060160586 ) ) ;
#7883=VERTEX_POINT ( 'NONE', #10522 ) ;
#7884=DIRECTION ( 'NONE',  ( 0.000000000000000000, -1.000000000000000000, -7.930164461608263644E-17 ) ) ;
#7889=ADVANCED_FACE ( 'NONE', ( #9357 ), #9296, .F. ) ;
#7890=DIRECTION ( 'NONE',  ( -1.000000000000000000, -0.000000000000000000, -0.000000000000000000 ) ) ;
#7892=EDGE_CURVE ( 'NONE', #10902, #11947, #9437, .T. ) ;
#7898=DIRECTION ( 'NONE',  ( 0.000000000000000000, -1.156482317317870246E-16, 1.000000000000000000 ) ) ;
#7909=DIRECTION ( 'NONE',  ( 0.000000000000000000, 0.000000000000000000, 1.000000000000000000 ) ) ;
#7910=CARTESIAN_POINT ( 'NONE',  ( -87.04832655144203102, 0.000000000000000000, -217.9289243767376831 ) ) ;
#7916=DIRECTION ( 'NONE',  ( -0.000000000000000000, 1.000000000000000000, 0.000000000000000000 ) ) ;
#7923=EDGE_LOOP ( 'NONE', ( #3540, #8900, #8474, #2649 ) ) ;
#7926=CARTESIAN_POINT ( 'NONE',  ( 1.249585401188644101E-12, 12.00000000000000000, 1.078643762690514762 ) ) ;
#7934=DIRECTION ( 'NONE',  ( 0.000000000000000000, 1.000000000000000000, 0.000000000000000000 ) ) ;
#7939=CARTESIAN_POINT ( 'NONE',  ( 35.00000000000000000, 81.99999999999998579, 272.3192290001959464 ) ) ;
#7942=EDGE_LOOP ( 'NONE', ( #10259, #3867, #8871, #6926 ) ) ;
#7946=DIRECTION ( 'NONE',  ( -0.000000000000000000, -1.000000000000000000, -0.000000000000000000 ) ) ;
#7951=VECTOR ( 'NONE', #1264, 1000.000000000000000 ) ;
#7953=ORIENTED_EDGE ( 'NONE', *, *, #5756, .T. ) ;
#7954=CARTESIAN_POINT ( 'NONE',  ( 126.4213562373094959, 12.00000000000000000, -6.938893903907228378E-15 ) ) ;
#7955=DIRECTION ( 'NONE',  ( 1.000000000000000000, 0.000000000000000000, 0.000000000000000000 ) ) ;
#7956=ADVANCED_FACE ( 'NONE', ( #8384 ), #3729, .F. ) ;
#7960=DIRECTION ( 'NONE',  ( -0.000000000000000000, -7.930164461608263644E-17, 1.000000000000000000 ) ) ;
#7962=DIRECTION ( 'NONE',  ( 0.000000000000000000, 0.000000000000000000, -1.000000000000000000 ) ) ;
#7967=AXIS2_PLACEMENT_3D ( 'NONE', #6712, #7579, #2891 ) ;
#7976=DIRECTION ( 'NONE',  ( 0.000000000000000000, -1.156482317317870246E-16, 1.000000000000000000 ) ) ;
#7979=ORIENTED_EDGE ( 'NONE', *, *, #7723, .F. ) ;
#7987=DIRECTION ( 'NONE',  ( 0.000000000000000000, 0.000000000000000000, 1.000000000000000000 ) ) ;
#7989=ADVANCED_FACE ( 'NONE', ( #2743 ), #9420, .F. ) ;
#7996=AXIS2_PLACEMENT_3D ( 'NONE', #5215, #6099, #450 ) ;
#7997=AXIS2_PLACEMENT_3D ( 'NONE', #3036, #6806, #431 ) ;
#8021=CARTESIAN_POINT ( 'NONE',  ( -35.00000000000000000, 0.000000000000000000, 190.3192290001959464 ) ) ;
#8027=FACE_BOUND ( 'NONE', #10846, .T. ) ;
#8028=DIRECTION ( 'NONE',  ( 0.000000000000000000, 0.000000000000000000, 1.000000000000000000 ) ) ;
#8033=CARTESIAN_POINT ( 'NONE',  ( -87.04832655144203102, 0.000000000000000000, -225.4289243767377116 ) ) ;
#8035=CARTESIAN_POINT ( 'NONE',  ( -151.3258811035894098, 0.000000000000000000, -48.63263083939678921 ) ) ;
#8038=CARTESIAN_POINT ( 'NONE',  ( 1.387778780781445676E-14, 163.9999999999999716, 126.4213562373094959 ) ) ;
#8039=EDGE_CURVE ( 'NONE', #83, #10273, #422, .T. ) ;
#8042=EDGE_LOOP ( 'NONE', ( #10969, #2366 ) ) ;
#8044=ORIENTED_EDGE ( 'NONE', *, *, #6177, .T. ) ;
#8049=DIRECTION ( 'NONE',  ( 0.000000000000000000, 0.000000000000000000, -1.000000000000000000 ) ) ;
#8052=ORIENTED_EDGE ( 'NONE', *, *, #2543, .T. ) ;
#8063=CIRCLE ( 'NONE', #2736, 7.500000000000007994 ) ;
#8066=EDGE_CURVE ( 'NONE', #9472, #7241, #11643, .T. ) ;
#8069=DIRECTION ( 'NONE',  ( -0.000000000000000000, 1.000000000000000000, 0.000000000000000000 ) ) ;
#8072=DIRECTION ( 'NONE',  ( 0.000000000000000000, -1.156482317317870246E-16, 1.000000000000000000 ) ) ;
#8074=VERTEX_POINT ( 'NONE', #7740 ) ;
#8077=DIRECTION ( 'NONE',  ( 0.000000000000000000, 0.000000000000000000, 1.000000000000000000 ) ) ;
#8085=DIRECTION ( 'NONE',  ( 0.000000000000000000, -1.156482317317870246E-16, 1.000000000000000000 ) ) ;
#8089=FACE_BOUND ( 'NONE', #10827, .T. ) ;
#8091=CIRCLE ( 'NONE', #3747, 7.500000000000007105 ) ;
#8093=CYLINDRICAL_SURFACE ( 'NONE', #362, 7.500000000000007105 ) ;
#8101=DIRECTION ( 'NONE',  ( 0.000000000000000000, 0.000000000000000000, -1.000000000000000000 ) ) ;
#8109=CYLINDRICAL_SURFACE ( 'NONE', #12004, 7.499999999999978684 ) ;
#8110=ORIENTED_EDGE ( 'NONE', *, *, #9929, .F. ) ;
#8117=ORIENTED_EDGE ( 'NONE', *, *, #4276, .F. ) ;
#8118=DIRECTION ( 'NONE',  ( 0.000000000000000000, 1.000000000000000000, 0.000000000000000000 ) ) ;
#8119=LINE ( 'NONE', #7882, #4610 ) ;
#8126=AXIS2_PLACEMENT_3D ( 'NONE', #4087, #6864, #6055 ) ;
#8127=DIRECTION ( 'NONE',  ( -0.000000000000000000, -1.000000000000000000, -0.000000000000000000 ) ) ;
#8132=CYLINDRICAL_SURFACE ( 'NONE', #3628, 7.500000000000007105 ) ;
#8137=EDGE_CURVE ( 'NONE', #2477, #6316, #4279, .T. ) ;
#8142=CARTESIAN_POINT ( 'NONE',  ( 35.00000000000000000, 81.99999999999998579, 190.3192290001959748 ) ) ;
#8143=DIRECTION ( 'NONE',  ( 0.000000000000000000, 0.000000000000000000, -1.000000000000000000 ) ) ;
#8144=FACE_BOUND ( 'NONE', #10995, .T. ) ;
#8145=CARTESIAN_POINT ( 'NONE',  ( 0.000000000000000000, 0.000000000000000000, -89.68077099980401101 ) ) ;
#8148=ORIENTED_EDGE ( 'NONE', *, *, #3877, .T. ) ;
#8152=CARTESIAN_POINT ( 'NONE',  ( -35.00000000000000000, 81.99999999999998579, 260.3192290001960032 ) ) ;
#8153=DIRECTION ( 'NONE',  ( -0.000000000000000000, -1.000000000000000000, -0.000000000000000000 ) ) ;
#8156=EDGE_LOOP ( 'NONE', ( #687, #9011 ) ) ;
#8161=DIRECTION ( 'NONE',  ( 0.000000000000000000, -0.000000000000000000, 1.000000000000000000 ) ) ;
#8163=CARTESIAN_POINT ( 'NONE',  ( 9.371890508914830252E-13, 152.0000000000000000, -36.42135623730948168 ) ) ;
#8165=DIRECTION ( 'NONE',  ( 0.000000000000000000, -1.156482317317870246E-16, 1.000000000000000000 ) ) ;
#8168=AXIS2_PLACEMENT_3D ( 'NONE', #9739, #7833, #7898 ) ;
#8173=ADVANCED_FACE ( 'NONE', ( #7113 ), #8109, .F. ) ;
#8174=ORIENTED_EDGE ( 'NONE', *, *, #1452, .T. ) ;
#8176=DIRECTION ( 'NONE',  ( 0.000000000000000000, 0.000000000000000000, 1.000000000000000000 ) ) ;
#8180=ORIENTED_EDGE ( 'NONE', *, *, #6565, .T. ) ;
#8185=CIRCLE ( 'NONE', #2865, 7.500000000000013323 ) ;
#8187=CYLINDRICAL_SURFACE ( 'NONE', #7007, 7.500000000000007105 ) ;
#8191=DIRECTION ( 'NONE',  ( -0.000000000000000000, -1.000000000000000000, -0.000000000000000000 ) ) ;
#8192=CARTESIAN_POINT ( 'NONE',  ( 6.247927005943220505E-13, 0.000000000000000000, -66.42135623730949590 ) ) ;
#8194=MANIFOLD_SOLID_BREP ( 'Cut-Extrude5', #1181 ) ;
#8198=CIRCLE ( 'NONE', #2874, 7.500000000000007105 ) ;
#8200=ORIENTED_EDGE ( 'NONE', *, *, #2583, .T. ) ;
#8208=DIRECTION ( 'NONE',  ( -0.000000000000000000, -1.000000000000000000, -0.000000000000000000 ) ) ;
#8212=CARTESIAN_POINT ( 'NONE',  ( 1.249585401188644101E-12, -6.000000000000006217, 1.078643762690512986 ) ) ;
#8213=EDGE_CURVE ( 'NONE', #8695, #11947, #560, .T. ) ;
#8218=ORIENTED_EDGE ( 'NONE', *, *, #6770, .F. ) ;
#8221=ADVANCED_FACE ( 'NONE', ( #11860 ), #12046, .F. ) ;
#8223=CARTESIAN_POINT ( 'NONE',  ( -120.8820948793972434, 0.000000000000000000, -194.1989091883324363 ) ) ;
#8226=EDGE_LOOP ( 'NONE', ( #6800, #11713 ) ) ;
#8227=EDGE_LOOP ( 'NONE', ( #4043, #2623, #6297, #8963 ) ) ;
#8229=EDGE_CURVE ( 'NONE', #11656, #11886, #1594, .T. ) ;
#8234=DIRECTION ( 'NONE',  ( 0.000000000000000000, 0.000000000000000000, 1.000000000000000000 ) ) ;
#8237=CYLINDRICAL_SURFACE ( 'NONE', #1683, 7.500000000000007105 ) ;
#8243=AXIS2_PLACEMENT_3D ( 'NONE', #6466, #7517, #9435 ) ;
#8245=VERTEX_POINT ( 'NONE', #605 ) ;
#8246=CYLINDRICAL_SURFACE ( 'NONE', #7456, 7.500000000000020428 ) ;
#8247=ORIENTED_EDGE ( 'NONE', *, *, #9069, .F. ) ;
#8256=CARTESIAN_POINT ( 'NONE',  ( 87.04832655144112152, 12.00000000000000000, -210.4289243767383368 ) ) ;
#8257=CARTESIAN_POINT ( 'NONE',  ( -144.0488662551579182, 12.00000000000000000, -139.4077238332691877 ) ) ;
#8264=COLOUR_RGB ( '', 0.31764706, 0.68627451, 0.89019608) ;
#8265=PLANE ( 'NONE',  #892 ) ;
#8271=EDGE_CURVE ( 'NONE', #7504, #4601, #1165, .T. ) ;
#8272=DIRECTION ( 'NONE',  ( -0.000000000000000000, -1.000000000000000000, -0.000000000000000000 ) ) ;
#8280=DIRECTION ( 'NONE',  ( 0.000000000000000000, 0.000000000000000000, 1.000000000000000000 ) ) ;
#8282=DIRECTION ( 'NONE',  ( 0.000000000000000000, 0.000000000000000000, 1.000000000000000000 ) ) ;
#8284=AXIS2_PLACEMENT_3D ( 'NONE', #7156, #4262, #8028 ) ;
#8288=DIRECTION ( 'NONE',  ( 0.000000000000000000, 0.000000000000000000, 1.000000000000000000 ) ) ;
#8289=CARTESIAN_POINT ( 'NONE',  ( -154.5043356068770493, 12.00000000000000000, -102.0666613060160302 ) ) ;
#8290=CYLINDRICAL_SURFACE ( 'NONE', #3640, 7.500000000000020428 ) ;
#8291=ADVANCED_FACE ( 'NONE', ( #670 ), #3374, .F. ) ;
#8293=VERTEX_POINT ( 'NONE', #9198 ) ;
#8298=CYLINDRICAL_SURFACE ( 'NONE', #10351, 7.500000000000007105 ) ;
#8306=CARTESIAN_POINT ( 'NONE',  ( 35.00000000000000000, 11.99999999999999289, 81.78351099501843180 ) ) ;
#8307=VERTEX_POINT ( 'NONE', #8223 ) ;
#8310=EDGE_CURVE ( 'NONE', #4288, #7231, #1538, .T. ) ;
#8317=VERTEX_POINT ( 'NONE', #3321 ) ;
#8320=ORIENTED_EDGE ( 'NONE', *, *, #235, .T. ) ;
#8322=FACE_OUTER_BOUND ( 'NONE', #2384, .T. ) ;
#8329=ORIENTED_EDGE ( 'NONE', *, *, #253, .F. ) ;
#8333=VERTEX_POINT ( 'NONE', #11919 ) ;
#8352=AXIS2_PLACEMENT_3D ( 'NONE', #6122, #11689, #3322 ) ;
#8355=ORIENTED_EDGE ( 'NONE', *, *, #6062, .F. ) ;
#8365=FACE_OUTER_BOUND ( 'NONE', #9975, .T. ) ;
#8366=VERTEX_POINT ( 'NONE', #3558 ) ;
#8372=ORIENTED_EDGE ( 'NONE', *, *, #9069, .T. ) ;
#8378=ADVANCED_FACE ( 'NONE', ( #10124 ), #1657, .F. ) ;
#8379=VECTOR ( 'NONE', #1779, 1000.000000000000000 ) ;
#8383=CARTESIAN_POINT ( 'NONE',  ( -35.00000000000000000, 81.99999999999998579, 190.3192290001959748 ) ) ;
#8384=FACE_OUTER_BOUND ( 'NONE', #4666, .T. ) ;
#8385=CARTESIAN_POINT ( 'NONE',  ( 154.5043356068769071, 12.00000000000000000, -94.56666130601712439 ) ) ;
#8387=CARTESIAN_POINT ( 'NONE',  ( -35.00000000000000000, 81.99999999999998579, 190.3192290001959748 ) ) ;
#8389=AXIS2_PLACEMENT_3D ( 'NONE', #10760, #420, #7987 ) ;
#8390=DIRECTION ( 'NONE',  ( 0.000000000000000000, 1.000000000000000000, 0.000000000000000000 ) ) ;
#8394=ORIENTED_EDGE ( 'NONE', *, *, #8749, .F. ) ;
#8407=AXIS2_PLACEMENT_3D ( 'NONE', #10391, #7554, #4776 ) ;
#8412=ORIENTED_EDGE ( 'NONE', *, *, #7262, .F. ) ;
#8430=DIRECTION ( 'NONE',  ( 0.000000000000000000, 0.000000000000000000, 1.000000000000000000 ) ) ;
#8431=EDGE_CURVE ( 'NONE', #8293, #4980, #9263, .T. ) ;
#8435=ADVANCED_FACE ( 'NONE', ( #12182 ), #11253, .F. ) ;
#8440=VERTEX_POINT ( 'NONE', #9391 ) ;
#8442=CARTESIAN_POINT ( 'NONE',  ( -151.3258811035894098, 12.00000000000000000, -48.63263083939678921 ) ) ;
#8444=DIRECTION ( 'NONE',  ( 0.000000000000000000, 0.000000000000000000, 1.000000000000000000 ) ) ;
#8446=DIRECTION ( 'NONE',  ( 0.000000000000000000, 0.000000000000000000, 1.000000000000000000 ) ) ;
#8447=VECTOR ( 'NONE', #10369, 1000.000000000000000 ) ;
#8452=CARTESIAN_POINT ( 'NONE',  ( -120.8820948793972434, 12.00000000000000000, -186.6989091883324363 ) ) ;
#8453=AXIS2_PLACEMENT_3D ( 'NONE', #10043, #9173, #7260 ) ;
#8459=CYLINDRICAL_SURFACE ( 'NONE', #7789, 7.500000000000007105 ) ;
#8461=ORIENTED_EDGE ( 'NONE', *, *, #9229, .T. ) ;
#8467=EDGE_CURVE ( 'NONE', #10476, #1493, #8063, .T. ) ;
#8469=CARTESIAN_POINT ( 'NONE',  ( 1.249585401188644101E-12, -6.000000000000005329, -6.421356237309495008 ) ) ;
#8471=ORIENTED_EDGE ( 'NONE', *, *, #7723, .T. ) ;
#8474=ORIENTED_EDGE ( 'NONE', *, *, #11897, .F. ) ;
#8478=VECTOR ( 'NONE', #11404, 1000.000000000000000 ) ;
#8479=ORIENTED_EDGE ( 'NONE', *, *, #1932, .F. ) ;
#8482=DIRECTION ( 'NONE',  ( -0.000000000000000000, 1.189524669241239115E-16, -1.000000000000000000 ) ) ;
#8486=DIRECTION ( 'NONE',  ( -1.000000000000000000, -0.000000000000000000, -0.000000000000000000 ) ) ;
#8489=ORIENTED_EDGE ( 'NONE', *, *, #4478, .T. ) ;
#8504=DIRECTION ( 'NONE',  ( 0.000000000000000000, 0.000000000000000000, 1.000000000000000000 ) ) ;
#8508=EDGE_CURVE ( 'NONE', #8781, #6173, #10435, .T. ) ;
#8510=ORIENTED_EDGE ( 'NONE', *, *, #11988, .T. ) ;
#8514=ORIENTED_EDGE ( 'NONE', *, *, #9932, .F. ) ;
#8520=EDGE_LOOP ( 'NONE', ( #11581, #10010 ) ) ;
#8524=EDGE_CURVE ( 'NONE', #694, #2733, #9443, .T. ) ;
#8525=VERTEX_POINT ( 'NONE', #2839 ) ;
#8527=LINE ( 'NONE', #4864, #6057 ) ;
#8528=CARTESIAN_POINT ( 'NONE',  ( -35.00000000000000000, 163.9999999999999716, 190.3192290001959748 ) ) ;
#8531=VERTEX_POINT ( 'NONE', #8528 ) ;
#8532=DIRECTION ( 'NONE',  ( 0.000000000000000000, 1.000000000000000000, 0.000000000000000000 ) ) ;
#8537=CARTESIAN_POINT ( 'NONE',  ( 120.8820948793965186, 12.00000000000000000, -194.1989091883332890 ) ) ;
#8539=CIRCLE ( 'NONE', #3191, 7.500000000000007105 ) ;
#8540=VERTEX_POINT ( 'NONE', #6421 ) ;
#8546=DIRECTION ( 'NONE',  ( 0.000000000000000000, 1.000000000000000000, 0.000000000000000000 ) ) ;
#8556=EDGE_CURVE ( 'NONE', #5849, #7221, #5492, .T. ) ;
#8557=DIRECTION ( 'NONE',  ( -0.000000000000000000, -1.000000000000000000, -0.000000000000000000 ) ) ;
#8562=ORIENTED_EDGE ( 'NONE', *, *, #1998, .T. ) ;
#8564=CARTESIAN_POINT ( 'NONE',  ( 9.371890508914830252E-13, -6.000000000000006217, -28.92135623730948524 ) ) ;
#8577=AXIS2_PLACEMENT_3D ( 'NONE', #4919, #7524, #216 ) ;
#8585=AXIS2_PLACEMENT_3D ( 'NONE', #9674, #9225, #766 ) ;
#8588=ORIENTED_EDGE ( 'NONE', *, *, #2496, .F. ) ;
#8592=EDGE_CURVE ( 'NONE', #6719, #4553, #1290, .T. ) ;
#8593=AXIS2_PLACEMENT_3D ( 'NONE', #6401, #5054, #10172 ) ;
#8595=CIRCLE ( 'NONE', #11754, 7.500000000000013323 ) ;
#8597=EDGE_LOOP ( 'NONE', ( #5433, #8200 ) ) ;
#8598=LINE ( 'NONE', #11436, #1544 ) ;
#8601=FACE_BOUND ( 'NONE', #383, .T. ) ;
#8607=CARTESIAN_POINT ( 'NONE',  ( -126.4213562373094959, 0.000000000000000000, 2.255140518769849223E-14 ) ) ;
#8616=ORIENTED_EDGE ( 'NONE', *, *, #2543, .F. ) ;
#8629=ORIENTED_EDGE ( 'NONE', *, *, #8039, .F. ) ;
#8632=CARTESIAN_POINT ( 'NONE',  ( -126.4213562373094959, 12.00000000000000000, 2.255140518769849223E-14 ) ) ;
#8633=CARTESIAN_POINT ( 'NONE',  ( 35.00000000000000000, 11.99999999999998046, 190.3192290001959748 ) ) ;
#8635=AXIS2_PLACEMENT_3D ( 'NONE', #1976, #6371, #688 ) ;
#8638=FACE_OUTER_BOUND ( 'NONE', #9835, .T. ) ;
#8642=AXIS2_PLACEMENT_3D ( 'NONE', #409, #7916, #10861 ) ;
#8645=AXIS2_PLACEMENT_3D ( 'NONE', #3597, #707, #9040 ) ;
#8646=ORIENTED_EDGE ( 'NONE', *, *, #544, .T. ) ;
#8648=DIRECTION ( 'NONE',  ( -0.000000000000000000, 1.000000000000000000, 7.930164461608263644E-17 ) ) ;
#8650=ADVANCED_FACE ( 'NONE', ( #4073 ), #10734, .F. ) ;
#8653=EDGE_LOOP ( 'NONE', ( #4167, #1991, #9590, #4700 ) ) ;
#8656=CARTESIAN_POINT ( 'NONE',  ( 120.8820948793965186, 12.00000000000000000, -186.6989091883332890 ) ) ;
#8659=DIRECTION ( 'NONE',  ( 0.000000000000000000, 0.000000000000000000, 1.000000000000000000 ) ) ;
#8664=DIRECTION ( 'NONE',  ( 0.000000000000000000, 0.000000000000000000, -1.000000000000000000 ) ) ;
#8665=FACE_BOUND ( 'NONE', #9847, .T. ) ;
#8666=ORIENTED_EDGE ( 'NONE', *, *, #8965, .T. ) ;
#8670=ORIENTED_EDGE ( 'NONE', *, *, #6565, .F. ) ;
#8680=EDGE_CURVE ( 'NONE', #2603, #6447, #3944, .T. ) ;
#8682=ORIENTED_EDGE ( 'NONE', *, *, #9843, .F. ) ;
#8683=ORIENTED_EDGE ( 'NONE', *, *, #9499, .F. ) ;
#8687=AXIS2_PLACEMENT_3D ( 'NONE', #8469, #4434, #7275 ) ;
#8695=VERTEX_POINT ( 'NONE', #348 ) ;
#8697=CYLINDRICAL_SURFACE ( 'NONE', #6939, 7.500000000000007105 ) ;
#8702=CYLINDRICAL_SURFACE ( 'NONE', #1650, 7.500000000000007105 ) ;
#8703=ORIENTED_EDGE ( 'NONE', *, *, #9458, .T. ) ;
#8709=ORIENTED_EDGE ( 'NONE', *, *, #7667, .F. ) ;
#8712=CARTESIAN_POINT ( 'NONE',  ( 35.00000000000000000, 2.428612866367529932E-14, -159.6807709998040252 ) ) ;
#8717=VERTEX_POINT ( 'NONE', #3189 ) ;
#8721=FACE_BOUND ( 'NONE', #601, .T. ) ;
#8724=ORIENTED_EDGE ( 'NONE', *, *, #10993, .T. ) ;
#8725=AXIS2_PLACEMENT_3D ( 'NONE', #7910, #4870, #9632 ) ;
#8726=CARTESIAN_POINT ( 'NONE',  ( 2.186774452080127126E-12, -6.000000000000006217, 91.07864376269050410 ) ) ;
#8729=CIRCLE ( 'NONE', #4000, 7.500000000000007105 ) ;
#8734=DIRECTION ( 'NONE',  ( 0.000000000000000000, 1.000000000000000000, 0.000000000000000000 ) ) ;
#8747=CIRCLE ( 'NONE', #11894, 7.500000000000007105 ) ;
#8749=EDGE_CURVE ( 'NONE', #1654, #8525, #2943, .T. ) ;
#8753=CARTESIAN_POINT ( 'NONE',  ( -35.00000000000000000, 152.0000000000000000, -124.6807709998038689 ) ) ;
#8761=AXIS2_PLACEMENT_3D ( 'NONE', #9983, #3299, #8072 ) ;
#8780=LINE ( 'NONE', #6736, #9520 ) ;
#8781=VERTEX_POINT ( 'NONE', #9745 ) ;
#8782=VERTEX_POINT ( 'NONE', #10467 ) ;
#8783=CIRCLE ( 'NONE', #2275, 7.500000000000013323 ) ;
#8787=EDGE_LOOP ( 'NONE', ( #8514, #277, #3621, #5369 ) ) ;
#8788=ADVANCED_FACE ( 'NONE', ( #6253 ), #3275, .F. ) ;
#8792=EDGE_CURVE ( 'NONE', #9472, #10481, #3731, .T. ) ;
#8793=CARTESIAN_POINT ( 'NONE',  ( 0.000000000000000000, 12.00000000000000000, -264.6807709998040536 ) ) ;
#8797=EDGE_CURVE ( 'NONE', #10145, #4052, #3000, .T. ) ;
#8800=EDGE_LOOP ( 'NONE', ( #9907, #7779 ) ) ;
#8805=ORIENTED_EDGE ( 'NONE', *, *, #3976, .T. ) ;
#8807=ORIENTED_EDGE ( 'NONE', *, *, #2581, .T. ) ;
#8809=EDGE_CURVE ( 'NONE', #10118, #7042, #6704, .T. ) ;
#8820=CIRCLE ( 'NONE', #4289, 35.00000000000002842 ) ;
#8822=ORIENTED_EDGE ( 'NONE', *, *, #10394, .F. ) ;
#8825=CARTESIAN_POINT ( 'NONE',  ( 1.561981751485805177E-12, -6.000000000000005329, 23.57864376269050410 ) ) ;
#8826=LINE ( 'NONE', #9749, #9604 ) ;
#8828=CIRCLE ( 'NONE', #1335, 7.500000000000007105 ) ;
#8832=ORIENTED_EDGE ( 'NONE', *, *, #11394, .T. ) ;
#8835=CARTESIAN_POINT ( 'NONE',  ( 126.4213562373094959, 0.000000000000000000, -6.938893903907228378E-15 ) ) ;
#8837=CARTESIAN_POINT ( 'NONE',  ( -87.04832655144203102, 12.00000000000000000, -217.9289243767376831 ) ) ;
#8849=CARTESIAN_POINT ( 'NONE',  ( 0.000000000000000000, 12.00000000000000000, -89.68077099980401101 ) ) ;
#8851=VECTOR ( 'NONE', #421, 1000.000000000000000 ) ;
#8853=ADVANCED_FACE ( 'NONE', ( #2475 ), #7176, .F. ) ;
#8856=DIRECTION ( 'NONE',  ( -0.000000000000000000, -1.000000000000000000, -0.000000000000000000 ) ) ;
#8867=EDGE_CURVE ( 'NONE', #10381, #2733, #11818, .T. ) ;
#8871=ORIENTED_EDGE ( 'NONE', *, *, #4356, .T. ) ;
#8874=CARTESIAN_POINT ( 'NONE',  ( -35.00000000000000000, 163.9999999999999716, 190.3192290001959748 ) ) ;
#8885=VERTEX_POINT ( 'NONE', #8306 ) ;
#8886=DIRECTION ( 'NONE',  ( -0.000000000000000000, -1.000000000000000000, -0.000000000000000000 ) ) ;
#8888=CARTESIAN_POINT ( 'NONE',  ( -120.8820948793972434, 12.00000000000000000, -194.1989091883324363 ) ) ;
#8891=ORIENTED_EDGE ( 'NONE', *, *, #9101, .T. ) ;
#8892=CIRCLE ( 'NONE', #3972, 7.500000000000007105 ) ;
#8897=EDGE_LOOP ( 'NONE', ( #5855, #11069 ) ) ;
#8899=AXIS2_PLACEMENT_3D ( 'NONE', #777, #11960, #11228 ) ;
#8900=ORIENTED_EDGE ( 'NONE', *, *, #8524, .T. ) ;
#8907=ORIENTED_EDGE ( 'NONE', *, *, #2654, .T. ) ;
#8910=ORIENTED_EDGE ( 'NONE', *, *, #9478, .F. ) ;
#8911=CIRCLE ( 'NONE', #848, 7.500000000000007105 ) ;
#8914=DIRECTION ( 'NONE',  ( -0.000000000000000000, 1.189524669241239115E-16, -1.000000000000000000 ) ) ;
#8916=DIRECTION ( 'NONE',  ( 0.000000000000000000, 1.000000000000000000, 0.000000000000000000 ) ) ;
#8919=CARTESIAN_POINT ( 'NONE',  ( 126.4213562373094959, 0.000000000000000000, -6.938893903907228378E-15 ) ) ;
#8925=EDGE_CURVE ( 'NONE', #7221, #11989, #7489, .T. ) ;
#8926=CARTESIAN_POINT ( 'NONE',  ( 6.247927005943220505E-13, 164.0000000000000000, -66.42135623730948168 ) ) ;
#8930=EDGE_CURVE ( 'NONE', #2603, #8317, #9838, .T. ) ;
#8934=CARTESIAN_POINT ( 'NONE',  ( -126.4213562373094959, 12.00000000000000000, -7.499999999999991118 ) ) ;
#8938=ORIENTED_EDGE ( 'NONE', *, *, #2907, .T. ) ;
#8942=CARTESIAN_POINT ( 'NONE',  ( -87.04832655144203102, 12.00000000000000000, -225.4289243767377116 ) ) ;
#8943=AXIS2_PLACEMENT_3D ( 'NONE', #7954, #10790, #10668 ) ;
#8945=VECTOR ( 'NONE', #5133, 1000.000000000000000 ) ;
#8946=DIRECTION ( 'NONE',  ( -1.000000000000000000, -0.000000000000000000, -0.000000000000000000 ) ) ;
#8952=EDGE_CURVE ( 'NONE', #6215, #338, #4529, .T. ) ;
#8955=CIRCLE ( 'NONE', #3627, 7.500000000000007105 ) ;
#8963=ORIENTED_EDGE ( 'NONE', *, *, #10141, .T. ) ;
#8965=EDGE_CURVE ( 'NONE', #125, #5383, #11630, .T. ) ;
#8967=AXIS2_PLACEMENT_3D ( 'NONE', #5629, #939, #749 ) ;
#8971=FACE_OUTER_BOUND ( 'NONE', #9009, .T. ) ;
#8984=FACE_OUTER_BOUND ( 'NONE', #10275, .T. ) ;
#8989=CARTESIAN_POINT ( 'NONE',  ( 87.04832655144112152, 12.00000000000000000, -217.9289243767383368 ) ) ;
#8990=ORIENTED_EDGE ( 'NONE', *, *, #11746, .F. ) ;
#8999=FACE_BOUND ( 'NONE', #8156, .T. ) ;
#9001=CIRCLE ( 'NONE', #2492, 175.0000000000000000 ) ;
#9009=EDGE_LOOP ( 'NONE', ( #45, #7369, #10494, #5898 ) ) ;
#9011=ORIENTED_EDGE ( 'NONE', *, *, #11971, .F. ) ;
#9013=FACE_BOUND ( 'NONE', #2726, .T. ) ;
#9019=DIRECTION ( 'NONE',  ( 0.000000000000000000, 1.000000000000000000, 0.000000000000000000 ) ) ;
#9023=ORIENTED_EDGE ( 'NONE', *, *, #10458, .T. ) ;
#9026=AXIS2_PLACEMENT_3D ( 'NONE', #2003, #4837, #2985 ) ;
#9031=DIRECTION ( 'NONE',  ( -0.000000000000000000, 1.000000000000000000, 0.000000000000000000 ) ) ;
#9034=AXIS2_PLACEMENT_3D ( 'NONE', #9585, #3895, #6797 ) ;
#9038=CARTESIAN_POINT ( 'NONE',  ( -87.04832655144203102, 0.000000000000000000, -217.9289243767376831 ) ) ;
#9040=DIRECTION ( 'NONE',  ( 0.000000000000000000, 0.000000000000000000, -1.000000000000000000 ) ) ;
#9041=APPLICATION_CONTEXT ( 'automotive_design' ) ;
#9042=CIRCLE ( 'NONE', #2354, 175.0000000000000000 ) ;
#9048=CARTESIAN_POINT ( 'NONE',  ( 0.000000000000000000, 0.000000000000000000, 0.000000000000000000 ) ) ;
#9051=DIRECTION ( 'NONE',  ( 0.000000000000000000, 0.000000000000000000, 1.000000000000000000 ) ) ;
#9056=LINE ( 'NONE', #10177, #5283 ) ;
#9062=CARTESIAN_POINT ( 'NONE',  ( -35.00000000000000000, 11.99999999999999822, 40.70327710424895429 ) ) ;
#9063=DIRECTION ( 'NONE',  ( -0.000000000000000000, 1.000000000000000000, 7.930164461608263644E-17 ) ) ;
#9066=FACE_OUTER_BOUND ( 'NONE', #2609, .T. ) ;
#9069=EDGE_CURVE ( 'NONE', #8317, #2603, #4720, .T. ) ;
#9070=DIRECTION ( 'NONE',  ( -0.000000000000000000, 1.000000000000000000, 0.000000000000000000 ) ) ;
#9072=DIRECTION ( 'NONE',  ( -0.000000000000000000, 1.000000000000000000, -0.000000000000000000 ) ) ;
#9076=FACE_OUTER_BOUND ( 'NONE', #9937, .T. ) ;
#9077=FACE_BOUND ( 'NONE', #8226, .T. ) ;
#9084=ORIENTED_EDGE ( 'NONE', *, *, #6765, .F. ) ;
#9091=CARTESIAN_POINT ( 'NONE',  ( -144.0488662551579182, 12.00000000000000000, -146.9077238332691877 ) ) ;
#9097=EDGE_CURVE ( 'NONE', #5849, #9567, #8598, .T. ) ;
#9099=AXIS2_PLACEMENT_3D ( 'NONE', #10501, #4933, #1117 ) ;
#9101=EDGE_CURVE ( 'NONE', #11989, #9567, #7874, .T. ) ;
#9108=ADVANCED_FACE ( 'NONE', ( #6118 ), #8093, .F. ) ;
#9109=AXIS2_PLACEMENT_3D ( 'NONE', #734, #10990, #8288 ) ;
#9113=CARTESIAN_POINT ( 'NONE',  ( 3.123963502971610252E-13, 12.00000000000000000, -96.42135623730949590 ) ) ;
#9114=ORIENTED_EDGE ( 'NONE', *, *, #7451, .T. ) ;
#9128=CARTESIAN_POINT ( 'NONE',  ( -126.4213562373094959, 12.00000000000000000, 7.500000000000036415 ) ) ;
#9133=DIRECTION ( 'NONE',  ( -1.000000000000000000, -0.000000000000000000, 0.000000000000000000 ) ) ;
#9135=EDGE_LOOP ( 'NONE', ( #11885, #4411 ) ) ;
#9136=CIRCLE ( 'NONE', #871, 7.500000000000007105 ) ;
#9142=DIRECTION ( 'NONE',  ( 0.000000000000000000, 1.000000000000000000, 0.000000000000000000 ) ) ;
#9145=DIRECTION ( 'NONE',  ( -0.000000000000000000, 1.000000000000000000, 7.930164461608263644E-17 ) ) ;
#9157=DIRECTION ( 'NONE',  ( -0.000000000000000000, 1.000000000000000000, -0.000000000000000000 ) ) ;
#9158=EDGE_CURVE ( 'NONE', #2533, #10730, #2127, .T. ) ;
#9162=ORIENTED_EDGE ( 'NONE', *, *, #1269, .F. ) ;
#9169=FACE_OUTER_BOUND ( 'NONE', #11181, .T. ) ;
#9171=DIRECTION ( 'NONE',  ( 0.000000000000000000, 0.000000000000000000, 1.000000000000000000 ) ) ;
#9173=DIRECTION ( 'NONE',  ( 0.000000000000000000, 1.000000000000000000, 0.000000000000000000 ) ) ;
#9179=EDGE_CURVE ( 'NONE', #5557, #7042, #6465, .T. ) ;
#9184=CARTESIAN_POINT ( 'NONE',  ( 45.53315400109643463, 0.000000000000000000, -245.3419396193597493 ) ) ;
#9188=FACE_OUTER_BOUND ( 'NONE', #10642, .T. ) ;
#9189=LINE ( 'NONE', #8212, #11921 ) ;
#9198=CARTESIAN_POINT ( 'NONE',  ( 2.187692937179487324E-12, 152.0000000000000000, 76.07864376269050410 ) ) ;
#9202=PRODUCT_DEFINITION_FORMATION_WITH_SPECIFIED_SOURCE ( 'ANY', '', #4767, .NOT_KNOWN. ) ;
#9223=VERTEX_POINT ( 'NONE', #8035 ) ;
#9224=AXIS2_PLACEMENT_3D ( 'NONE', #10164, #4549, #7388 ) ;
#9225=DIRECTION ( 'NONE',  ( -0.000000000000000000, -1.000000000000000000, -0.000000000000000000 ) ) ;
#9229=EDGE_CURVE ( 'NONE', #6316, #5191, #11793, .T. ) ;
#9232=DIRECTION ( 'NONE',  ( 0.000000000000000000, 0.000000000000000000, 1.000000000000000000 ) ) ;
#9236=CARTESIAN_POINT ( 'NONE',  ( 6.247927005943220505E-13, 164.0000000000000000, -58.92135623730947458 ) ) ;
#9237=CARTESIAN_POINT ( 'NONE',  ( 154.5043356068769071, 0.000000000000000000, -94.56666130601712439 ) ) ;
#9241=CARTESIAN_POINT ( 'NONE',  ( 1.874378101782966050E-12, -6.000000000000005329, 53.57864376269050410 ) ) ;
#9245=DIRECTION ( 'NONE',  ( 0.000000000000000000, 1.000000000000000000, 0.000000000000000000 ) ) ;
#9248=DIRECTION ( 'NONE',  ( -0.000000000000000000, -1.000000000000000000, -0.000000000000000000 ) ) ;
#9250=VECTOR ( 'NONE', #5943, 1000.000000000000000 ) ;
#9259=ORIENTED_EDGE ( 'NONE', *, *, #1847, .T. ) ;
#9263=LINE ( 'NONE', #4639, #10631 ) ;
#9264=DIRECTION ( 'NONE',  ( -0.000000000000000000, -1.000000000000000000, -0.000000000000000000 ) ) ;
#9268=AXIS2_PLACEMENT_3D ( 'NONE', #11307, #1664, #10315 ) ;
#9284=ORIENTED_EDGE ( 'NONE', *, *, #2615, .F. ) ;
#9288=EDGE_CURVE ( 'NONE', #10860, #4714, #2456, .T. ) ;
#9289=ORIENTED_EDGE ( 'NONE', *, *, #7892, .F. ) ;
#9296=PLANE ( 'NONE',  #9026 ) ;
#9305=ORIENTED_EDGE ( 'NONE', *, *, #11520, .F. ) ;
#9309=EDGE_LOOP ( 'NONE', ( #827, #8666 ) ) ;
#9310=DIRECTION ( 'NONE',  ( 0.000000000000000000, 0.000000000000000000, 1.000000000000000000 ) ) ;
#9312=DIRECTION ( 'NONE',  ( -0.000000000000000000, -1.000000000000000000, -0.000000000000000000 ) ) ;
#9315=FACE_OUTER_BOUND ( 'NONE', #1239, .T. ) ;
#9319=VECTOR ( 'NONE', #3190, 1000.000000000000000 ) ;
#9346=CIRCLE ( 'NONE', #1848, 7.500000000000007105 ) ;
#9347=EDGE_LOOP ( 'NONE', ( #11469, #1997, #10305, #7556 ) ) ;
#9354=ORIENTED_EDGE ( 'NONE', *, *, #4745, .F. ) ;
#9356=DIRECTION ( 'NONE',  ( 0.000000000000000000, 0.000000000000000000, -1.000000000000000000 ) ) ;
#9357=FACE_OUTER_BOUND ( 'NONE', #2776, .T. ) ;
#9359=CARTESIAN_POINT ( 'NONE',  ( 35.00000000000000000, 152.0000000000000000, 190.3192290001959748 ) ) ;
#9362=LINE ( 'NONE', #5391, #2113 ) ;
#9363=DIRECTION ( 'NONE',  ( 0.000000000000000000, 0.000000000000000000, -1.000000000000000000 ) ) ;
#9369=VERTEX_POINT ( 'NONE', #731 ) ;
#9375=ORIENTED_EDGE ( 'NONE', *, *, #1269, .T. ) ;
#9380=AXIS2_PLACEMENT_3D ( 'NONE', #2253, #5026, #5088 ) ;
#9391=CARTESIAN_POINT ( 'NONE',  ( 120.8820948793965186, 0.000000000000000000, -179.1989091883332890 ) ) ;
#9397=LINE ( 'NONE', #933, #6695 ) ;
#9403=CARTESIAN_POINT ( 'NONE',  ( -151.3258811035894098, 12.00000000000000000, -63.63263083939681053 ) ) ;
#9404=VERTEX_POINT ( 'NONE', #9128 ) ;
#9410=AXIS2_PLACEMENT_3D ( 'NONE', #2986, #11516, #2124 ) ;
#9413=DIRECTION ( 'NONE',  ( 0.000000000000000000, 1.000000000000000000, 0.000000000000000000 ) ) ;
#9420=CYLINDRICAL_SURFACE ( 'NONE', #6666, 7.500000000000007105 ) ;
#9422=DIRECTION ( 'NONE',  ( 0.000000000000000000, 1.000000000000000000, 0.000000000000000000 ) ) ;
#9435=DIRECTION ( 'NONE',  ( 0.000000000000000000, -1.156482317317870246E-16, 1.000000000000000000 ) ) ;
#9437=CIRCLE ( 'NONE', #4703, 7.500000000000020428 ) ;
#9443=CIRCLE ( 'NONE', #10816, 134.9999999999999716 ) ;
#9458=EDGE_CURVE ( 'NONE', #3054, #10902, #6577, .T. ) ;
#9459=LINE ( 'NONE', #2040, #5016 ) ;
#9461=FACE_OUTER_BOUND ( 'NONE', #3169, .T. ) ;
#9463=CIRCLE ( 'NONE', #11038, 7.500000000000007994 ) ;
#9464=FACE_BOUND ( 'NONE', #5692, .T. ) ;
#9472=VERTEX_POINT ( 'NONE', #3663 ) ;
#9475=DIRECTION ( 'NONE',  ( 0.000000000000000000, -1.156482317317870246E-16, 1.000000000000000000 ) ) ;
#9477=AXIS2_PLACEMENT_3D ( 'NONE', #1042, #3069, #7645 ) ;
#9478=EDGE_CURVE ( 'NONE', #10836, #3679, #9796, .T. ) ;
#9479=EDGE_CURVE ( 'NONE', #5900, #11808, #2488, .T. ) ;
#9480=DIRECTION ( 'NONE',  ( -0.000000000000000000, 1.000000000000000000, -0.000000000000000000 ) ) ;
#9484=DIRECTION ( 'NONE',  ( 0.000000000000000000, 1.000000000000000000, 0.000000000000000000 ) ) ;
#9486=ORIENTED_EDGE ( 'NONE', *, *, #544, .F. ) ;
#9491=ADVANCED_FACE ( 'NONE', ( #4038 ), #11579, .T. ) ;
#9495=CARTESIAN_POINT ( 'NONE',  ( -6.106226635438360972E-13, 12.00000000000000000, -252.1807709998039115 ) ) ;
#9497=CARTESIAN_POINT ( 'NONE',  ( 126.4213562373094959, 0.000000000000000000, -7.500000000000020428 ) ) ;
#9499=EDGE_CURVE ( 'NONE', #10559, #5214, #10648, .T. ) ;
#9505=ORIENTED_EDGE ( 'NONE', *, *, #4369, .T. ) ;
#9507=EDGE_CURVE ( 'NONE', #8317, #5359, #6819, .T. ) ;
#9510=AXIS2_PLACEMENT_3D ( 'NONE', #4146, #3204, #5128 ) ;
#9514=CARTESIAN_POINT ( 'NONE',  ( -144.0488662551579182, 12.00000000000000000, -154.4077238332691877 ) ) ;
#9519=EDGE_LOOP ( 'NONE', ( #1301, #3305 ) ) ;
#9520=VECTOR ( 'NONE', #7614, 1000.000000000000000 ) ;
#9523=DIRECTION ( 'NONE',  ( 0.000000000000000000, 0.000000000000000000, 1.000000000000000000 ) ) ;
#9524=ORIENTED_EDGE ( 'NONE', *, *, #9777, .T. ) ;
#9526=AXIS2_PLACEMENT_3D ( 'NONE', #5198, #9031, #572 ) ;
#9529=FACE_OUTER_BOUND ( 'NONE', #6738, .T. ) ;
#9531=ORIENTED_EDGE ( 'NONE', *, *, #3118, .F. ) ;
#9540=EDGE_CURVE ( 'NONE', #1863, #8366, #1087, .T. ) ;
#9550=ORIENTED_EDGE ( 'NONE', *, *, #5385, .F. ) ;
#9554=VECTOR ( 'NONE', #3909, 1000.000000000000000 ) ;
#9560=DIRECTION ( 'NONE',  ( 0.000000000000000000, 0.000000000000000000, 1.000000000000000000 ) ) ;
#9562=ADVANCED_FACE ( 'NONE', ( #2935 ), #7812, .T. ) ;
#9563=AXIS2_PLACEMENT_3D ( 'NONE', #5503, #6249, #5367 ) ;
#9567=VERTEX_POINT ( 'NONE', #2007 ) ;
#9571=AXIS2_PLACEMENT_3D ( 'NONE', #3953, #1861, #4017 ) ;
#9573=VERTEX_POINT ( 'NONE', #4960 ) ;
#9575=ADVANCED_FACE ( 'NONE', ( #254 ), #4787, .F. ) ;
#9581=AXIS2_PLACEMENT_3D ( 'NONE', #6828, #6947, #10533 ) ;
#9584=ORIENTED_EDGE ( 'NONE', *, *, #7454, .F. ) ;
#9585=CARTESIAN_POINT ( 'NONE',  ( 45.53315400109643463, 12.00000000000000000, -237.8419396193597208 ) ) ;
#9590=ORIENTED_EDGE ( 'NONE', *, *, #3405, .T. ) ;
#9591=DIRECTION ( 'NONE',  ( 0.000000000000000000, 0.000000000000000000, 1.000000000000000000 ) ) ;
#9593=ORIENTED_EDGE ( 'NONE', *, *, #3755, .T. ) ;
#9595=FACE_OUTER_BOUND ( 'NONE', #10173, .T. ) ;
#9604=VECTOR ( 'NONE', #5408, 1000.000000000000000 ) ;
#9610=EDGE_LOOP ( 'NONE', ( #11490, #2207 ) ) ;
#9612=ORIENTED_EDGE ( 'NONE', *, *, #5019, .T. ) ;
#9616=CARTESIAN_POINT ( 'NONE',  ( 35.00000000000000000, 152.0000000000000000, -124.6807709998038689 ) ) ;
#9617=CIRCLE ( 'NONE', #4091, 7.500000000000007994 ) ;
#9627=EDGE_CURVE ( 'NONE', #1702, #4714, #7232, .T. ) ;
#9630=ORIENTED_EDGE ( 'NONE', *, *, #8556, .F. ) ;
#9631=CARTESIAN_POINT ( 'NONE',  ( -126.4213562373094959, 12.00000000000000000, 2.255140518769849223E-14 ) ) ;
#9632=DIRECTION ( 'NONE',  ( 0.000000000000000000, 0.000000000000000000, 1.000000000000000000 ) ) ;
#9636=DIRECTION ( 'NONE',  ( 0.000000000000000000, 0.000000000000000000, 1.000000000000000000 ) ) ;
#9637=VECTOR ( 'NONE', #7960, 1000.000000000000000 ) ;
#9642=AXIS2_PLACEMENT_3D ( 'NONE', #10191, #12114, #5674 ) ;
#9644=EDGE_CURVE ( 'NONE', #8525, #1654, #11188, .T. ) ;
#9647=EDGE_LOOP ( 'NONE', ( #6375, #1109, #11556, #9305 ) ) ;
#9649=ORIENTED_EDGE ( 'NONE', *, *, #4133, .F. ) ;
#9653=EDGE_CURVE ( 'NONE', #6215, #2282, #10980, .T. ) ;
#9664=EDGE_LOOP ( 'NONE', ( #631, #1773, #8588, #1247 ) ) ;
#9665=DIRECTION ( 'NONE',  ( -0.000000000000000000, -1.000000000000000000, -0.000000000000000000 ) ) ;
#9670=VERTEX_POINT ( 'NONE', #9841 ) ;
#9674=CARTESIAN_POINT ( 'NONE',  ( 151.3258811035896656, 12.00000000000000000, -56.13263083939798292 ) ) ;
#9686=CARTESIAN_POINT ( 'NONE',  ( -87.04832655144203102, 12.00000000000000000, -210.4289243767376831 ) ) ;
#9691=CARTESIAN_POINT ( 'NONE',  ( -151.3258811035894098, 0.000000000000000000, -56.13263083939680342 ) ) ;
#9693=CARTESIAN_POINT ( 'NONE',  ( 9.381075359908434252E-13, 164.0000000000000000, -43.92135623730948879 ) ) ;
#9698=ORIENTED_EDGE ( 'NONE', *, *, #6443, .F. ) ;
#9706=AXIS2_PLACEMENT_3D ( 'NONE', #8825, #5224, #2389 ) ;
#9707=CARTESIAN_POINT ( 'NONE',  ( 6.247927005943220505E-13, 152.0000000000000000, -58.92135623730947458 ) ) ;
#9714=CIRCLE ( 'NONE', #6362, 7.500000000000020428 ) ;
#9724=ORIENTED_EDGE ( 'NONE', *, *, #1929, .T. ) ;
#9739=CARTESIAN_POINT ( 'NONE',  ( 2.186774452080127126E-12, -6.000000000000005329, 83.57864376269050410 ) ) ;
#9740=CIRCLE ( 'NONE', #7382, 7.500000000000007105 ) ;
#9743=ORIENTED_EDGE ( 'NONE', *, *, #10751, .F. ) ;
#9745=CARTESIAN_POINT ( 'NONE',  ( 2.186774452080127126E-12, 152.0000000000000000, 91.07864376269051832 ) ) ;
#9746=DIRECTION ( 'NONE',  ( -0.000000000000000000, 1.000000000000000000, 7.930164461608263644E-17 ) ) ;
#9747=CIRCLE ( 'NONE', #11733, 7.500000000000007105 ) ;
#9749=CARTESIAN_POINT ( 'NONE',  ( 126.4213562373094959, 12.00000000000000000, -7.500000000000020428 ) ) ;
#9757=AXIS2_PLACEMENT_3D ( 'NONE', #6428, #7298, #1665 ) ;
#9759=EDGE_CURVE ( 'NONE', #11886, #4553, #3278, .T. ) ;
#9761=CARTESIAN_POINT ( 'NONE',  ( 144.0488662551573782, 0.000000000000000000, -139.4077238332702109 ) ) ;
#9763=CARTESIAN_POINT ( 'NONE',  ( 9.381075359908434252E-13, -6.000000000000004441, -43.92135623730950300 ) ) ;
#9771=DIRECTION ( 'NONE',  ( 0.000000000000000000, 0.000000000000000000, -1.000000000000000000 ) ) ;
#9773=CARTESIAN_POINT ( 'NONE',  ( 35.00000000000000000, 81.99999999999998579, 190.3192290001959748 ) ) ;
#9776=VERTEX_POINT ( 'NONE', #1389 ) ;
#9777=EDGE_CURVE ( 'NONE', #4285, #64, #2429, .T. ) ;
#9779=EDGE_LOOP ( 'NONE', ( #6869, #11216, #6644, #10222 ) ) ;
#9787=DIRECTION ( 'NONE',  ( 0.000000000000000000, 0.000000000000000000, 1.000000000000000000 ) ) ;
#9794=ADVANCED_FACE ( 'NONE', ( #1507 ), #3404, .F. ) ;
#9796=CIRCLE ( 'NONE', #9410, 7.500000000000007105 ) ;
#9809=CARTESIAN_POINT ( 'NONE',  ( -35.00000000000000000, 2.428612866367529932E-14, -159.6807709998040252 ) ) ;
#9814=FACE_BOUND ( 'NONE', #4582, .T. ) ;
#9816=CARTESIAN_POINT ( 'NONE',  ( 0.000000000000000000, 164.0000000000000000, -126.4213562373094959 ) ) ;
#9823=DIRECTION ( 'NONE',  ( -0.000000000000000000, 1.000000000000000000, 7.930164461608263644E-17 ) ) ;
#9825=EDGE_CURVE ( 'NONE', #1640, #3716, #3473, .T. ) ;
#9828=ORIENTED_EDGE ( 'NONE', *, *, #4033, .T. ) ;
#9833=CARTESIAN_POINT ( 'NONE',  ( 3.123963502971610252E-13, -6.000000000000006217, -88.92135623730948168 ) ) ;
#9835=EDGE_LOOP ( 'NONE', ( #8683, #10776, #8489, #5730 ) ) ;
#9838=CIRCLE ( 'NONE', #7047, 7.500000000000007105 ) ;
#9841=CARTESIAN_POINT ( 'NONE',  ( 1.387778780781445676E-14, 0.000000000000000000, 133.9213562373095101 ) ) ;
#9843=EDGE_CURVE ( 'NONE', #4515, #10844, #9617, .T. ) ;
#9846=EDGE_CURVE ( 'NONE', #9369, #6223, #3285, .T. ) ;
#9847=EDGE_LOOP ( 'NONE', ( #6994, #9114, #9162, #8832, #9883 ) ) ;
#9861=FACE_OUTER_BOUND ( 'NONE', #7923, .T. ) ;
#9863=VERTEX_POINT ( 'NONE', #3472 ) ;
#9868=ADVANCED_FACE ( 'NONE', ( #8322 ), #6389, .F. ) ;
#9874=CARTESIAN_POINT ( 'NONE',  ( -87.04832655144203102, 12.00000000000000000, -217.9289243767376831 ) ) ;
#9875=EDGE_CURVE ( 'NONE', #8333, #8717, #6256, .T. ) ;
#9883=ORIENTED_EDGE ( 'NONE', *, *, #7463, .T. ) ;
#9886=CARTESIAN_POINT ( 'NONE',  ( 2.187692937179487324E-12, 163.9999999999999716, 76.07864376269050410 ) ) ;
#9889=DIRECTION ( 'NONE',  ( 0.000000000000000000, 1.000000000000000000, 0.000000000000000000 ) ) ;
#9896=DIRECTION ( 'NONE',  ( -0.000000000000000000, -1.000000000000000000, -0.000000000000000000 ) ) ;
#9900=ORIENTED_EDGE ( 'NONE', *, *, #7359, .T. ) ;
#9904=ORIENTED_EDGE ( 'NONE', *, *, #3877, .F. ) ;
#9907=ORIENTED_EDGE ( 'NONE', *, *, #2893, .F. ) ;
#9912=CARTESIAN_POINT ( 'NONE',  ( 35.00000000000000000, 12.00000000000000000, 40.70327710424895429 ) ) ;
#9913=ADVANCED_FACE ( 'NONE', ( #5524 ), #12153, .F. ) ;
#9921=DIRECTION ( 'NONE',  ( 0.000000000000000000, 0.000000000000000000, 1.000000000000000000 ) ) ;
#9922=EDGE_LOOP ( 'NONE', ( #10093, #6946 ) ) ;
#9929=EDGE_CURVE ( 'NONE', #11819, #9863, #11955, .T. ) ;
#9931=AXIS2_PLACEMENT_3D ( 'NONE', #473, #10808, #4268 ) ;
#9932=EDGE_CURVE ( 'NONE', #8245, #5183, #5851, .T. ) ;
#9933=FACE_BOUND ( 'NONE', #3876, .T. ) ;
#9937=EDGE_LOOP ( 'NONE', ( #7065, #2464, #3218, #5513 ) ) ;
#9942=DIRECTION ( 'NONE',  ( 0.000000000000000000, 0.000000000000000000, 1.000000000000000000 ) ) ;
#9944=VECTOR ( 'NONE', #3453, 1000.000000000000000 ) ;
#9946=EDGE_LOOP ( 'NONE', ( #6260, #1845, #6602, #1004 ) ) ;
#9947=EDGE_CURVE ( 'NONE', #5383, #125, #12187, .T. ) ;
#9949=FACE_OUTER_BOUND ( 'NONE', #11614, .T. ) ;
#9951=CARTESIAN_POINT ( 'NONE',  ( 45.53315400109643463, 12.00000000000000000, -245.3419396193597493 ) ) ;
#9954=DIRECTION ( 'NONE',  ( 0.000000000000000000, 0.000000000000000000, 1.000000000000000000 ) ) ;
#9956=CIRCLE ( 'NONE', #5407, 7.500000000000007105 ) ;
#9960=EDGE_LOOP ( 'NONE', ( #6693, #5611, #6564, #3239 ) ) ;
#9963=VECTOR ( 'NONE', #6088, 1000.000000000000000 ) ;
#9967=EDGE_LOOP ( 'NONE', ( #8372, #1225, #11691, #5572 ) ) ;
#9975=EDGE_LOOP ( 'NONE', ( #8329, #452, #2229, #9531 ) ) ;
#9976=CARTESIAN_POINT ( 'NONE',  ( 126.4213562373094959, 12.00000000000000000, 7.500000000000007105 ) ) ;
#9981=EDGE_CURVE ( 'NONE', #8885, #2093, #9362, .T. ) ;
#9983=CARTESIAN_POINT ( 'NONE',  ( 9.371890508914830252E-13, -6.000000000000005329, -36.42135623730949590 ) ) ;
#9986=CARTESIAN_POINT ( 'NONE',  ( -35.00000000000000000, 164.0000000000000000, -124.6807709998038689 ) ) ;
#9987=ORIENTED_EDGE ( 'NONE', *, *, #8965, .F. ) ;
#9995=LINE ( 'NONE', #10739, #5301 ) ;
#9997=DIRECTION ( 'NONE',  ( 0.000000000000000000, -0.000000000000000000, 1.000000000000000000 ) ) ;
#9998=CARTESIAN_POINT ( 'NONE',  ( -144.0488662551579182, 0.000000000000000000, -139.4077238332691877 ) ) ;
#10005=FACE_OUTER_BOUND ( 'NONE', #7256, .T. ) ;
#10006=EDGE_CURVE ( 'NONE', #8885, #9472, #9001, .T. ) ;
#10010=ORIENTED_EDGE ( 'NONE', *, *, #2696, .F. ) ;
#10016=CARTESIAN_POINT ( 'NONE',  ( 35.00000000000000000, 12.00000000000002309, -159.6807709998040252 ) ) ;
#10021=EDGE_LOOP ( 'NONE', ( #8479, #2661, #7477, #8670 ) ) ;
#10023=VERTEX_POINT ( 'NONE', #2624 ) ;
#10024=ADVANCED_FACE ( 'NONE', ( #1709 ), #4743, .F. ) ;
#10038=AXIS2_PLACEMENT_3D ( 'NONE', #5370, #12061, #7364 ) ;
#10043=CARTESIAN_POINT ( 'NONE',  ( -154.5043356068770493, 12.00000000000000000, -102.0666613060160302 ) ) ;
#10045=EDGE_LOOP ( 'NONE', ( #10142, #7647, #10934, #5278 ) ) ;
#10055=CARTESIAN_POINT ( 'NONE',  ( 35.00000000000000000, 81.99999999999998579, 260.3192290001960032 ) ) ;
#10056=DIRECTION ( 'NONE',  ( 0.000000000000000000, 0.000000000000000000, 1.000000000000000000 ) ) ;
#10057=VECTOR ( 'NONE', #4498, 1000.000000000000000 ) ;
#10058=CARTESIAN_POINT ( 'NONE',  ( 126.4213562373094959, 12.00000000000000000, -6.938893903907228378E-15 ) ) ;
#10066=EDGE_CURVE ( 'NONE', #647, #4463, #6847, .T. ) ;
#10078=( NAMED_UNIT ( * ) PLANE_ANGLE_UNIT ( ) SI_UNIT ( $, .RADIAN. ) );
#10080=DIRECTION ( 'NONE',  ( -0.000000000000000000, -1.000000000000000000, -0.000000000000000000 ) ) ;
#10084=VECTOR ( 'NONE', #6212, 1000.000000000000000 ) ;
#10091=ORIENTED_EDGE ( 'NONE', *, *, #6698, .T. ) ;
#10093=ORIENTED_EDGE ( 'NONE', *, *, #7667, .T. ) ;
#10096=AXIS2_PLACEMENT_3D ( 'NONE', #1243, #411, #7856 ) ;
#10097=DIRECTION ( 'NONE',  ( -0.000000000000000000, 1.000000000000000000, -0.000000000000000000 ) ) ;
#10098=EDGE_CURVE ( 'NONE', #7181, #11998, #8820, .T. ) ;
#10110=CARTESIAN_POINT ( 'NONE',  ( 3.133148353965215262E-13, -6.000000000000004441, -103.9213562373094959 ) ) ;
#10114=AXIS2_PLACEMENT_3D ( 'NONE', #4802, #1964, #2199 ) ;
#10117=DIRECTION ( 'NONE',  ( 0.000000000000000000, 1.000000000000000000, 0.000000000000000000 ) ) ;
#10118=VERTEX_POINT ( 'NONE', #2537 ) ;
#10124=FACE_OUTER_BOUND ( 'NONE', #7821, .T. ) ;
#10129=EDGE_LOOP ( 'NONE', ( #11525, #4340, #8174, #1559 ) ) ;
#10134=EDGE_CURVE ( 'NONE', #4463, #4959, #8527, .T. ) ;
#10136=DIRECTION ( 'NONE',  ( 0.000000000000000000, 0.000000000000000000, 1.000000000000000000 ) ) ;
#10137=EDGE_LOOP ( 'NONE', ( #8938, #9023 ) ) ;
#10138=CARTESIAN_POINT ( 'NONE',  ( -45.53315400109751465, 12.00000000000000000, -237.8419396193594650 ) ) ;
#10140=( NAMED_UNIT ( * ) SI_UNIT ( $, .STERADIAN. ) SOLID_ANGLE_UNIT ( ) );
#10141=EDGE_CURVE ( 'NONE', #1000, #11268, #10434, .T. ) ;
#10142=ORIENTED_EDGE ( 'NONE', *, *, #2299, .F. ) ;
#10145=VERTEX_POINT ( 'NONE', #7310 ) ;
#10146=ORIENTED_EDGE ( 'NONE', *, *, #2447, .T. ) ;
#10149=DIRECTION ( 'NONE',  ( 0.000000000000000000, 0.000000000000000000, 1.000000000000000000 ) ) ;
#10154=ORIENTED_EDGE ( 'NONE', *, *, #1452, .F. ) ;
#10155=ADVANCED_FACE ( 'NONE', ( #157 ), #6312, .T. ) ;
#10156=ORIENTED_EDGE ( 'NONE', *, *, #5912, .T. ) ;
#10160=DIRECTION ( 'NONE',  ( -0.000000000000000000, 1.000000000000000000, -0.000000000000000000 ) ) ;
#10164=CARTESIAN_POINT ( 'NONE',  ( 144.0488662551573782, 0.000000000000000000, -146.9077238332702109 ) ) ;
#10165=DIRECTION ( 'NONE',  ( 0.000000000000000000, 1.000000000000000000, 0.000000000000000000 ) ) ;
#10172=DIRECTION ( 'NONE',  ( 0.000000000000000000, 0.000000000000000000, 1.000000000000000000 ) ) ;
#10173=EDGE_LOOP ( 'NONE', ( #9354, #8412, #8044, #4966 ) ) ;
#10174=ADVANCED_FACE ( 'NONE', ( #7592 ), #4810, .T. ) ;
#10176=EDGE_CURVE ( 'NONE', #6019, #11124, #11008, .T. ) ;
#10177=CARTESIAN_POINT ( 'NONE',  ( -35.00000000000000000, 12.00000000000002309, -159.6807709998040252 ) ) ;
#10178=FACE_OUTER_BOUND ( 'NONE', #8227, .T. ) ;
#10184=DIRECTION ( 'NONE',  ( -0.000000000000000000, 1.000000000000000000, 0.000000000000000000 ) ) ;
#10191=CARTESIAN_POINT ( 'NONE',  ( 1.561981751485805177E-12, 0.000000000000000000, 23.57864376269050410 ) ) ;
#10192=DIRECTION ( 'NONE',  ( 0.000000000000000000, 1.000000000000000000, 0.000000000000000000 ) ) ;
#10194=ORIENTED_EDGE ( 'NONE', *, *, #10176, .F. ) ;
#10195=ORIENTED_EDGE ( 'NONE', *, *, #5497, .T. ) ;
#10196=AXIS2_PLACEMENT_3D ( 'NONE', #9038, #10784, #11661 ) ;
#10198=LINE ( 'NONE', #7356, #1281 ) ;
#10204=CARTESIAN_POINT ( 'NONE',  ( 35.00000000000000000, 81.99999999999998579, 190.3192290001959748 ) ) ;
#10205=EDGE_LOOP ( 'NONE', ( #4815, #4005, #4838, #7609 ) ) ;
#10212=LINE ( 'NONE', #1749, #6749 ) ;
#10216=AXIS2_PLACEMENT_3D ( 'NONE', #299, #11744, #5988 ) ;
#10220=CARTESIAN_POINT ( 'NONE',  ( 1.249585401188644101E-12, 152.0000000000000000, -6.421356237309483461 ) ) ;
#10222=ORIENTED_EDGE ( 'NONE', *, *, #6177, .F. ) ;
#10223=CARTESIAN_POINT ( 'NONE',  ( 0.000000000000000000, -58.00000000000000711, -126.4213562373094959 ) ) ;
#10226=CARTESIAN_POINT ( 'NONE',  ( 1.387778780781445676E-14, 11.99999999999999645, 126.4213562373094959 ) ) ;
#10233=CIRCLE ( 'NONE', #7672, 7.500000000000007105 ) ;
#10236=FACE_OUTER_BOUND ( 'NONE', #2137, .T. ) ;
#10241=DIRECTION ( 'NONE',  ( 0.000000000000000000, -1.189524669241239115E-16, 1.000000000000000000 ) ) ;
#10248=CARTESIAN_POINT ( 'NONE',  ( 2.186774452080127126E-12, 12.00000000000000000, 83.57864376269050410 ) ) ;
#10254=VERTEX_POINT ( 'NONE', #4532 ) ;
#10259=ORIENTED_EDGE ( 'NONE', *, *, #5332, .F. ) ;
#10264=CARTESIAN_POINT ( 'NONE',  ( 1.874378101782966050E-12, 12.00000000000000000, 53.57864376269050410 ) ) ;
#10273=VERTEX_POINT ( 'NONE', #11967 ) ;
#10275=EDGE_LOOP ( 'NONE', ( #2637, #10195, #5329, #10326 ) ) ;
#10280=CARTESIAN_POINT ( 'NONE',  ( 151.3258811035896656, 0.000000000000000000, -48.63263083939796871 ) ) ;
#10285=DIRECTION ( 'NONE',  ( 0.000000000000000000, 0.000000000000000000, 1.000000000000000000 ) ) ;
#10289=EDGE_LOOP ( 'NONE', ( #4566, #11328 ) ) ;
#10290=CARTESIAN_POINT ( 'NONE',  ( 35.00000000000000000, 163.9999999999999716, 190.3192290001959748 ) ) ;
#10291=ADVANCED_FACE ( 'NONE', ( #10978 ), #11904, .F. ) ;
#10295=AXIS2_PLACEMENT_3D ( 'NONE', #7775, #1292, #4985 ) ;
#10299=LINE ( 'NONE', #6529, #2833 ) ;
#10305=ORIENTED_EDGE ( 'NONE', *, *, #11161, .T. ) ;
#10315=DIRECTION ( 'NONE',  ( 0.000000000000000000, 0.000000000000000000, -1.000000000000000000 ) ) ;
#10319=AXIS2_PLACEMENT_3D ( 'NONE', #2742, #5582, #9356 ) ;
#10326=ORIENTED_EDGE ( 'NONE', *, *, #8797, .F. ) ;
#10327=EDGE_CURVE ( 'NONE', #9573, #10254, #11208, .T. ) ;
#10334=CARTESIAN_POINT ( 'NONE',  ( 0.000000000000000000, 0.000000000000000000, -118.9213562373094817 ) ) ;
#10337=ORIENTED_EDGE ( 'NONE', *, *, #1462, .T. ) ;
#10344=AXIS2_PLACEMENT_3D ( 'NONE', #2929, #2983, #9475 ) ;
#10345=DIRECTION ( 'NONE',  ( -0.000000000000000000, 1.000000000000000000, 0.000000000000000000 ) ) ;
#10351=AXIS2_PLACEMENT_3D ( 'NONE', #3506, #11126, #3635 ) ;
#10352=FACE_BOUND ( 'NONE', #2010, .T. ) ;
#10353=CIRCLE ( 'NONE', #5803, 7.500000000000007105 ) ;
#10359=DIRECTION ( 'NONE',  ( 0.000000000000000000, 0.000000000000000000, -1.000000000000000000 ) ) ;
#10362=CIRCLE ( 'NONE', #9581, 7.500000000000007105 ) ;
#10364=ORIENTED_EDGE ( 'NONE', *, *, #9947, .F. ) ;
#10369=DIRECTION ( 'NONE',  ( 0.000000000000000000, 0.000000000000000000, -1.000000000000000000 ) ) ;
#10370=DIRECTION ( 'NONE',  ( -0.000000000000000000, 1.000000000000000000, 7.930164461608263644E-17 ) ) ;
#10374=DIRECTION ( 'NONE',  ( 0.000000000000000000, 0.000000000000000000, 1.000000000000000000 ) ) ;
#10381=VERTEX_POINT ( 'NONE', #1517 ) ;
#10384=ORIENTED_EDGE ( 'NONE', *, *, #7505, .T. ) ;
#10388=AXIS2_PLACEMENT_3D ( 'NONE', #10472, #9665, #4731 ) ;
#10391=CARTESIAN_POINT ( 'NONE',  ( 0.000000000000000000, 0.000000000000000000, -124.6807709998040110 ) ) ;
#10394=EDGE_CURVE ( 'NONE', #7119, #3163, #6068, .T. ) ;
#10398=AXIS2_PLACEMENT_3D ( 'NONE', #10226, #11089, #9232 ) ;
#10403=DIRECTION ( 'NONE',  ( 0.000000000000000000, 1.000000000000000000, 0.000000000000000000 ) ) ;
#10405=CIRCLE ( 'NONE', #8645, 7.500000000000007105 ) ;
#10412=ORIENTED_EDGE ( 'NONE', *, *, #3295, .F. ) ;
#10421=CARTESIAN_POINT ( 'NONE',  ( -120.8820948793972434, 12.00000000000000000, -186.6989091883324363 ) ) ;
#10429=CARTESIAN_POINT ( 'NONE',  ( -6.097041784444755962E-13, 12.00000000000000000, -237.1807709998039115 ) ) ;
#10434=LINE ( 'NONE', #3817, #10794 ) ;
#10435=LINE ( 'NONE', #2712, #5284 ) ;
#10438=DIRECTION ( 'NONE',  ( 0.000000000000000000, 0.000000000000000000, 1.000000000000000000 ) ) ;
#10440=DIRECTION ( 'NONE',  ( 0.000000000000000000, 1.000000000000000000, 0.000000000000000000 ) ) ;
#10441=VECTOR ( 'NONE', #3141, 1000.000000000000000 ) ;
#10445=DIRECTION ( 'NONE',  ( 0.000000000000000000, 1.000000000000000000, 0.000000000000000000 ) ) ;
#10448=AXIS2_PLACEMENT_3D ( 'NONE', #3703, #5619, #4758 ) ;
#10449=DIRECTION ( 'NONE',  ( 0.000000000000000000, 1.000000000000000000, 0.000000000000000000 ) ) ;
#10455=CARTESIAN_POINT ( 'NONE',  ( -45.53315400109751465, 0.000000000000000000, -245.3419396193594650 ) ) ;
#10458=EDGE_CURVE ( 'NONE', #83, #1863, #2504, .T. ) ;
#10465=LINE ( 'NONE', #186, #3615 ) ;
#10467=CARTESIAN_POINT ( 'NONE',  ( 144.0488662551573782, 0.000000000000000000, -154.4077238332702393 ) ) ;
#10468=DIRECTION ( 'NONE',  ( 0.000000000000000000, 0.000000000000000000, 1.000000000000000000 ) ) ;
#10469=EDGE_CURVE ( 'NONE', #739, #725, #10405, .T. ) ;
#10470=ORIENTED_EDGE ( 'NONE', *, *, #7613, .T. ) ;
#10471=EDGE_CURVE ( 'NONE', #6669, #3591, #4483, .T. ) ;
#10472=CARTESIAN_POINT ( 'NONE',  ( 0.000000000000000000, 12.00000000000000000, -89.68077099980401101 ) ) ;
#10476=VERTEX_POINT ( 'NONE', #11157 ) ;
#10481=VERTEX_POINT ( 'NONE', #2862 ) ;
#10483=FACE_OUTER_BOUND ( 'NONE', #650, .T. ) ;
#10484=DIRECTION ( 'NONE',  ( 1.000000000000000000, 0.000000000000000000, -0.000000000000000000 ) ) ;
#10490=DIRECTION ( 'NONE',  ( 0.000000000000000000, 1.000000000000000000, 0.000000000000000000 ) ) ;
#10491=AXIS2_PLACEMENT_3D ( 'NONE', #599, #11911, #7217 ) ;
#10494=ORIENTED_EDGE ( 'NONE', *, *, #11459, .F. ) ;
#10496=CARTESIAN_POINT ( 'NONE',  ( 0.000000000000000000, 164.0000000000000000, -124.6807709998038405 ) ) ;
#10498=CIRCLE ( 'NONE', #8126, 7.500000000000007105 ) ;
#10500=ORIENTED_EDGE ( 'NONE', *, *, #10141, .F. ) ;
#10501=CARTESIAN_POINT ( 'NONE',  ( 9.371890508914830252E-13, 164.0000000000000000, -36.42135623730948168 ) ) ;
#10511=FACE_BOUND ( 'NONE', #4396, .T. ) ;
#10522=CARTESIAN_POINT ( 'NONE',  ( 151.3258811035896656, 0.000000000000000000, -63.63263083939799003 ) ) ;
#10524=ORIENTED_EDGE ( 'NONE', *, *, #10006, .T. ) ;
#10532=ORIENTED_EDGE ( 'NONE', *, *, #1932, .T. ) ;
#10533=DIRECTION ( 'NONE',  ( 0.000000000000000000, 0.000000000000000000, 1.000000000000000000 ) ) ;
#10538=AXIS2_PLACEMENT_3D ( 'NONE', #9631, #7599, #10374 ) ;
#10539=CARTESIAN_POINT ( 'NONE',  ( 9.371890508914830252E-13, -6.000000000000005329, -36.42135623730949590 ) ) ;
#10547=ORIENTED_EDGE ( 'NONE', *, *, #8137, .T. ) ;
#10548=CIRCLE ( 'NONE', #7997, 81.99999999999998579 ) ;
#10551=EDGE_CURVE ( 'NONE', #64, #10481, #5154, .T. ) ;
#10557=AXIS2_PLACEMENT_3D ( 'NONE', #1658, #9133, #671 ) ;
#10559=VERTEX_POINT ( 'NONE', #7829 ) ;
#10562=DIRECTION ( 'NONE',  ( 0.000000000000000000, 1.000000000000000000, 0.000000000000000000 ) ) ;
#10570=ORIENTED_EDGE ( 'NONE', *, *, #9179, .F. ) ;
#10572=CARTESIAN_POINT ( 'NONE',  ( 35.00000000000000000, 81.99999999999998579, 190.3192290001959748 ) ) ;
#10578=CARTESIAN_POINT ( 'NONE',  ( 1.874378101782966050E-12, 163.9999999999999716, 61.07864376269052542 ) ) ;
#10591=CARTESIAN_POINT ( 'NONE',  ( 35.00000000000000000, 0.000000000000000000, 40.70327710424895429 ) ) ;
#10598=ORIENTED_EDGE ( 'NONE', *, *, #2496, .T. ) ;
#10604=CARTESIAN_POINT ( 'NONE',  ( 6.247927005943220505E-13, 0.000000000000000000, -58.92135623730948879 ) ) ;
#10609=VERTEX_POINT ( 'NONE', #2617 ) ;
#10610=DIRECTION ( 'NONE',  ( -0.000000000000000000, -1.000000000000000000, -0.000000000000000000 ) ) ;
#10614=DIRECTION ( 'NONE',  ( 0.000000000000000000, 0.000000000000000000, 1.000000000000000000 ) ) ;
#10615=EDGE_CURVE ( 'NONE', #5971, #1440, #3897, .T. ) ;
#10624=VECTOR ( 'NONE', #8272, 1000.000000000000000 ) ;
#10628=ORIENTED_EDGE ( 'NONE', *, *, #11356, .T. ) ;
#10631=VECTOR ( 'NONE', #987, 1000.000000000000000 ) ;
#10632=CYLINDRICAL_SURFACE ( 'NONE', #12084, 7.500000000000007105 ) ;
#10633=FACE_BOUND ( 'NONE', #5399, .T. ) ;
#10634=ORIENTED_EDGE ( 'NONE', *, *, #4942, .T. ) ;
#10637=ORIENTED_EDGE ( 'NONE', *, *, #6665, .F. ) ;
#10642=EDGE_LOOP ( 'NONE', ( #7636, #3493, #3099, #7845 ) ) ;
#10644=AXIS2_PLACEMENT_3D ( 'NONE', #6431, #7301, #879 ) ;
#10648=LINE ( 'NONE', #3919, #6836 ) ;
#10653=EDGE_LOOP ( 'NONE', ( #2498, #11710, #1433, #4451 ) ) ;
#10656=EDGE_LOOP ( 'NONE', ( #5200, #9698, #2954, #63 ) ) ;
#10657=CARTESIAN_POINT ( 'NONE',  ( 0.000000000000000000, 0.000000000000000000, -126.4213562373094959 ) ) ;
#10660=EDGE_LOOP ( 'NONE', ( #4702, #3772 ) ) ;
#10667=ORIENTED_EDGE ( 'NONE', *, *, #3264, .T. ) ;
#10668=DIRECTION ( 'NONE',  ( 0.000000000000000000, 0.000000000000000000, 1.000000000000000000 ) ) ;
#10676=DIRECTION ( 'NONE',  ( 0.000000000000000000, -1.000000000000000000, -7.930164461608263644E-17 ) ) ;
#10681=CARTESIAN_POINT ( 'NONE',  ( -35.00000000000000000, 12.00000000000000000, 40.70327710424895429 ) ) ;
#10682=EDGE_CURVE ( 'NONE', #2378, #4910, #8828, .T. ) ;
#10684=DIRECTION ( 'NONE',  ( 0.000000000000000000, 1.000000000000000000, 0.000000000000000000 ) ) ;
#10688=CYLINDRICAL_SURFACE ( 'NONE', #11687, 7.500000000000007994 ) ;
#10690=CARTESIAN_POINT ( 'NONE',  ( -154.5043356068770493, 0.000000000000000000, -102.0666613060160302 ) ) ;
#10692=CARTESIAN_POINT ( 'NONE',  ( 126.4213562373094959, 12.00000000000000000, -6.938893903907228378E-15 ) ) ;
#10728=CARTESIAN_POINT ( 'NONE',  ( 35.00000000000000000, 0.000000000000000000, 190.3192290001959464 ) ) ;
#10730=VERTEX_POINT ( 'NONE', #11959 ) ;
#10734=CYLINDRICAL_SURFACE ( 'NONE', #6492, 7.500000000000007105 ) ;
#10736=CIRCLE ( 'NONE', #8577, 7.500000000000007105 ) ;
#10739=CARTESIAN_POINT ( 'NONE',  ( 151.3258811035896656, 12.00000000000000000, -63.63263083939799003 ) ) ;
#10745=EDGE_LOOP ( 'NONE', ( #9584, #8682, #7043, #8805 ) ) ;
#10751=EDGE_CURVE ( 'NONE', #8782, #4959, #3694, .T. ) ;
#10760=CARTESIAN_POINT ( 'NONE',  ( 1.561981751485805177E-12, 152.0000000000000000, 23.57864376269051832 ) ) ;
#10767=ORIENTED_EDGE ( 'NONE', *, *, #10837, .T. ) ;
#10769=ADVANCED_FACE ( 'NONE', ( #8971 ), #8246, .F. ) ;
#10772=ORIENTED_EDGE ( 'NONE', *, *, #10976, .T. ) ;
#10776=ORIENTED_EDGE ( 'NONE', *, *, #6901, .F. ) ;
#10780=ORIENTED_EDGE ( 'NONE', *, *, #9158, .T. ) ;
#10784=DIRECTION ( 'NONE',  ( 0.000000000000000000, 1.000000000000000000, 0.000000000000000000 ) ) ;
#10790=DIRECTION ( 'NONE',  ( 0.000000000000000000, 1.000000000000000000, 0.000000000000000000 ) ) ;
#10794=VECTOR ( 'NONE', #5373, 1000.000000000000000 ) ;
#10801=FACE_BOUND ( 'NONE', #8520, .T. ) ;
#10808=DIRECTION ( 'NONE',  ( 0.000000000000000000, -1.000000000000000000, -7.930164461608263644E-17 ) ) ;
#10811=VECTOR ( 'NONE', #4156, 1000.000000000000000 ) ;
#10813=ORIENTED_EDGE ( 'NONE', *, *, #11458, .F. ) ;
#10815=LINE ( 'NONE', #1487, #5802 ) ;
#10816=AXIS2_PLACEMENT_3D ( 'NONE', #7534, #7594, #4577 ) ;
#10823=ORIENTED_EDGE ( 'NONE', *, *, #11154, .F. ) ;
#10827=EDGE_LOOP ( 'NONE', ( #7979, #9904 ) ) ;
#10828=ADVANCED_FACE ( 'NONE', ( #9529 ), #7733, .T. ) ;
#10832=CIRCLE ( 'NONE', #571, 7.500000000000007105 ) ;
#10836=VERTEX_POINT ( 'NONE', #10578 ) ;
#10837=EDGE_CURVE ( 'NONE', #4751, #2076, #3048, .T. ) ;
#10839=AXIS2_PLACEMENT_3D ( 'NONE', #10264, #2845, #1738 ) ;
#10844=VERTEX_POINT ( 'NONE', #11507 ) ;
#10846=EDGE_LOOP ( 'NONE', ( #12138, #6098 ) ) ;
#10847=DIRECTION ( 'NONE',  ( 0.000000000000000000, 1.000000000000000000, 0.000000000000000000 ) ) ;
#10852=EDGE_CURVE ( 'NONE', #5780, #2194, #10548, .T. ) ;
#10856=DIRECTION ( 'NONE',  ( 0.000000000000000000, 1.000000000000000000, 0.000000000000000000 ) ) ;
#10860=VERTEX_POINT ( 'NONE', #319 ) ;
#10861=DIRECTION ( 'NONE',  ( 0.000000000000000000, 0.000000000000000000, 1.000000000000000000 ) ) ;
#10865=DIRECTION ( 'NONE',  ( 0.000000000000000000, 1.000000000000000000, 0.000000000000000000 ) ) ;
#10869=AXIS2_PLACEMENT_3D ( 'NONE', #1280, #1392, #4173 ) ;
#10873=ORIENTED_EDGE ( 'NONE', *, *, #8952, .T. ) ;
#10880=VERTEX_POINT ( 'NONE', #4107 ) ;
#10883=CARTESIAN_POINT ( 'NONE',  ( 87.04832655144112152, 12.00000000000000000, -217.9289243767383368 ) ) ;
#10890=ORIENTED_EDGE ( 'NONE', *, *, #2427, .F. ) ;
#10892=CIRCLE ( 'NONE', #5573, 7.500000000000007105 ) ;
#10893=ORIENTED_EDGE ( 'NONE', *, *, #8508, .T. ) ;
#10894=AXIS2_PLACEMENT_3D ( 'NONE', #7287, #2579, #6351 ) ;
#10902=VERTEX_POINT ( 'NONE', #9237 ) ;
#10904=DIRECTION ( 'NONE',  ( 0.000000000000000000, 0.000000000000000000, 1.000000000000000000 ) ) ;
#10909=DIRECTION ( 'NONE',  ( 0.000000000000000000, 1.000000000000000000, 0.000000000000000000 ) ) ;
#10910=ORIENTED_EDGE ( 'NONE', *, *, #1319, .F. ) ;
#10913=AXIS2_PLACEMENT_3D ( 'NONE', #663, #12038, #2573 ) ;
#10918=CARTESIAN_POINT ( 'NONE',  ( 1.561981751485805177E-12, 0.000000000000000000, 23.57864376269050410 ) ) ;
#10922=FACE_BOUND ( 'NONE', #626, .T. ) ;
#10923=DIRECTION ( 'NONE',  ( 0.000000000000000000, 0.000000000000000000, -1.000000000000000000 ) ) ;
#10925=DIRECTION ( 'NONE',  ( 0.000000000000000000, 0.000000000000000000, 1.000000000000000000 ) ) ;
#10932=VECTOR ( 'NONE', #3639, 1000.000000000000000 ) ;
#10934=ORIENTED_EDGE ( 'NONE', *, *, #235, .F. ) ;
#10935=ORIENTED_EDGE ( 'NONE', *, *, #6698, .F. ) ;
#10941=CIRCLE ( 'NONE', #5613, 7.500000000000020428 ) ;
#10951=ORIENTED_EDGE ( 'NONE', *, *, #468, .T. ) ;
#10952=CIRCLE ( 'NONE', #8593, 7.500000000000007994 ) ;
#10955=DIRECTION ( 'NONE',  ( 0.000000000000000000, 0.000000000000000000, -1.000000000000000000 ) ) ;
#10956=ORIENTED_EDGE ( 'NONE', *, *, #12209, .T. ) ;
#10960=AXIS2_PLACEMENT_3D ( 'NONE', #8989, #4306, #8077 ) ;
#10961=EDGE_LOOP ( 'NONE', ( #4174, #3454, #9284, #11979 ) ) ;
#10965=DIRECTION ( 'NONE',  ( -0.000000000000000000, 1.000000000000000000, 7.930164461608263644E-17 ) ) ;
#10969=ORIENTED_EDGE ( 'NONE', *, *, #2857, .F. ) ;
#10976=EDGE_CURVE ( 'NONE', #10559, #1936, #9956, .T. ) ;
#10977=CARTESIAN_POINT ( 'NONE',  ( 120.8820948793965186, 12.00000000000000000, -179.1989091883332890 ) ) ;
#10978=FACE_OUTER_BOUND ( 'NONE', #6487, .T. ) ;
#10980=CIRCLE ( 'NONE', #3675, 7.500000000000007105 ) ;
#10981=FACE_OUTER_BOUND ( 'NONE', #6412, .T. ) ;
#10983=DIRECTION ( 'NONE',  ( 0.000000000000000000, 0.000000000000000000, 1.000000000000000000 ) ) ;
#10984=CARTESIAN_POINT ( 'NONE',  ( -154.5043356068770493, 0.000000000000000000, -102.0666613060160302 ) ) ;
#10985=FACE_BOUND ( 'NONE', #11034, .T. ) ;
#10990=DIRECTION ( 'NONE',  ( 0.000000000000000000, 1.000000000000000000, 0.000000000000000000 ) ) ;
#10991=DIRECTION ( 'NONE',  ( -0.000000000000000000, 1.000000000000000000, 7.930164461608263644E-17 ) ) ;
#10993=EDGE_CURVE ( 'NONE', #931, #10118, #6796, .T. ) ;
#10995=EDGE_LOOP ( 'NONE', ( #5963, #5257 ) ) ;
#11002=LINE ( 'NONE', #4456, #10932 ) ;
#11004=EDGE_LOOP ( 'NONE', ( #6886, #1271, #4903, #10813 ) ) ;
#11007=EDGE_LOOP ( 'NONE', ( #12107, #11637, #8394, #2187 ) ) ;
#11008=LINE ( 'NONE', #2838, #8447 ) ;
#11014=LINE ( 'NONE', #5378, #4228 ) ;
#11026=DIRECTION ( 'NONE',  ( 0.000000000000000000, 1.000000000000000000, 0.000000000000000000 ) ) ;
#11033=DIRECTION ( 'NONE',  ( 0.000000000000000000, 0.000000000000000000, 1.000000000000000000 ) ) ;
#11034=EDGE_LOOP ( 'NONE', ( #7008, #8218 ) ) ;
#11038=AXIS2_PLACEMENT_3D ( 'NONE', #1122, #4873, #8659 ) ;
#11048=FACE_OUTER_BOUND ( 'NONE', #344, .T. ) ;
#11054=DIRECTION ( 'NONE',  ( -0.000000000000000000, 1.000000000000000000, 0.000000000000000000 ) ) ;
#11058=EDGE_LOOP ( 'NONE', ( #5351, #3954, #3525, #7545 ) ) ;
#11061=FACE_OUTER_BOUND ( 'NONE', #3756, .T. ) ;
#11066=DIRECTION ( 'NONE',  ( 0.000000000000000000, 0.000000000000000000, 1.000000000000000000 ) ) ;
#11067=DIRECTION ( 'NONE',  ( 0.000000000000000000, 1.000000000000000000, 0.000000000000000000 ) ) ;
#11069=ORIENTED_EDGE ( 'NONE', *, *, #1131, .F. ) ;
#11072=EDGE_LOOP ( 'NONE', ( #10951, #1579 ) ) ;
#11075=VERTEX_POINT ( 'NONE', #3119 ) ;
#11079=ADVANCED_FACE ( 'NONE', ( #7762 ), #94, .F. ) ;
#11083=CARTESIAN_POINT ( 'NONE',  ( -154.5043356068770493, 12.00000000000000000, -109.5666613060160586 ) ) ;
#11086=ORIENTED_EDGE ( 'NONE', *, *, #8213, .F. ) ;
#11087=CARTESIAN_POINT ( 'NONE',  ( 6.257111856936825515E-13, -6.000000000000004441, -73.92135623730949590 ) ) ;
#11089=DIRECTION ( 'NONE',  ( 0.000000000000000000, 1.000000000000000000, 0.000000000000000000 ) ) ;
#11100=EDGE_LOOP ( 'NONE', ( #435, #5638 ) ) ;
#11102=CARTESIAN_POINT ( 'NONE',  ( 9.184850993605161750E-16, 0.000000000000000000, -133.9213562373095101 ) ) ;
#11106=CARTESIAN_POINT ( 'NONE',  ( 1.479627290717497352E-14, -58.00000000000000711, 118.9213562373094817 ) ) ;
#11116=ORIENTED_EDGE ( 'NONE', *, *, #6619, .F. ) ;
#11124=VERTEX_POINT ( 'NONE', #8753 ) ;
#11126=DIRECTION ( 'NONE',  ( -0.000000000000000000, -1.000000000000000000, -0.000000000000000000 ) ) ;
#11132=DIRECTION ( 'NONE',  ( 0.000000000000000000, 0.000000000000000000, 1.000000000000000000 ) ) ;
#11133=VERTEX_POINT ( 'NONE', #5032 ) ;
#11141=ORIENTED_EDGE ( 'NONE', *, *, #3584, .T. ) ;
#11143=AXIS2_PLACEMENT_3D ( 'NONE', #3267, #5304, #8161 ) ;
#11144=EDGE_CURVE ( 'NONE', #7589, #6019, #4801, .T. ) ;
#11149=DIRECTION ( 'NONE',  ( 0.000000000000000000, 1.000000000000000000, 0.000000000000000000 ) ) ;
#11152=VECTOR ( 'NONE', #6792, 1000.000000000000000 ) ;
#11154=EDGE_CURVE ( 'NONE', #8531, #11075, #4045, .T. ) ;
#11155=DIRECTION ( 'NONE',  ( 0.000000000000000000, 0.000000000000000000, 1.000000000000000000 ) ) ;
#11157=CARTESIAN_POINT ( 'NONE',  ( 1.249585401188644101E-12, 152.0000000000000000, 1.078643762690525199 ) ) ;
#11161=EDGE_CURVE ( 'NONE', #2093, #6037, #11659, .T. ) ;
#11165=FACE_BOUND ( 'NONE', #4240, .T. ) ;
#11181=EDGE_LOOP ( 'NONE', ( #10637, #2715, #7409, #6464 ) ) ;
#11184=DIRECTION ( 'NONE',  ( -0.000000000000000000, -1.000000000000000000, -0.000000000000000000 ) ) ;
#11188=CIRCLE ( 'NONE', #1317, 7.500000000000007105 ) ;
#11190=DIRECTION ( 'NONE',  ( -0.000000000000000000, 1.000000000000000000, 7.930164461608263644E-17 ) ) ;
#11195=VECTOR ( 'NONE', #8914, 1000.000000000000000 ) ;
#11204=DIRECTION ( 'NONE',  ( -0.000000000000000000, -1.000000000000000000, -0.000000000000000000 ) ) ;
#11208=CIRCLE ( 'NONE', #11788, 7.500000000000007105 ) ;
#11210=EDGE_LOOP ( 'NONE', ( #4845, #1992, #2945, #3182 ) ) ;
#11216=ORIENTED_EDGE ( 'NONE', *, *, #4745, .T. ) ;
#11219=CYLINDRICAL_SURFACE ( 'NONE', #10319, 7.500000000000013323 ) ;
#11224=CARTESIAN_POINT ( 'NONE',  ( 6.247927005943220505E-13, 152.0000000000000000, -66.42135623730948168 ) ) ;
#11228=DIRECTION ( 'NONE',  ( 0.000000000000000000, 0.000000000000000000, 1.000000000000000000 ) ) ;
#11232=( GEOMETRIC_REPRESENTATION_CONTEXT ( 3 ) GLOBAL_UNCERTAINTY_ASSIGNED_CONTEXT ( ( #6955 ) ) GLOBAL_UNIT_ASSIGNED_CONTEXT ( ( #1676, #10078, #10140 ) ) REPRESENTATION_CONTEXT ( 'NONE', 'WORKASPACE' ) );
#11236=EDGE_LOOP ( 'NONE', ( #241, #8646, #7137, #6381 ) ) ;
#11243=AXIS2_PLACEMENT_3D ( 'NONE', #5135, #3387, #8049 ) ;
#11244=CARTESIAN_POINT ( 'NONE',  ( 1.874378101782966050E-12, -6.000000000000006217, 61.07864376269051121 ) ) ;
#11253=CYLINDRICAL_SURFACE ( 'NONE', #6485, 7.500000000000007105 ) ;
#11257=EDGE_LOOP ( 'NONE', ( #5272, #6100 ) ) ;
#11268=VERTEX_POINT ( 'NONE', #9912 ) ;
#11278=DIRECTION ( 'NONE',  ( 0.000000000000000000, 0.000000000000000000, -1.000000000000000000 ) ) ;
#11279=CARTESIAN_POINT ( 'NONE',  ( 45.53315400109643463, 12.00000000000000000, -237.8419396193597208 ) ) ;
#11290=EDGE_CURVE ( 'NONE', #11808, #5900, #278, .T. ) ;
#11294=EDGE_LOOP ( 'NONE', ( #3702, #1807, #748, #4393 ) ) ;
#11297=ORIENTED_EDGE ( 'NONE', *, *, #9288, .T. ) ;
#11305=VERTEX_POINT ( 'NONE', #11889 ) ;
#11307=CARTESIAN_POINT ( 'NONE',  ( 154.5043356068769071, 12.00000000000000000, -102.0666613060171386 ) ) ;
#11314=ORIENTED_EDGE ( 'NONE', *, *, #789, .F. ) ;
#11318=AXIS2_PLACEMENT_3D ( 'NONE', #5482, #10184, #8282 ) ;
#11323=DIRECTION ( 'NONE',  ( -0.000000000000000000, -1.000000000000000000, -0.000000000000000000 ) ) ;
#11328=ORIENTED_EDGE ( 'NONE', *, *, #9932, .T. ) ;
#11331=DIRECTION ( 'NONE',  ( 0.000000000000000000, 1.000000000000000000, 0.000000000000000000 ) ) ;
#11332=CIRCLE ( 'NONE', #461, 7.500000000000007105 ) ;
#11334=FACE_OUTER_BOUND ( 'NONE', #9664, .T. ) ;
#11338=LINE ( 'NONE', #7754, #7951 ) ;
#11339=EDGE_LOOP ( 'NONE', ( #6515, #7530, #10873, #1248 ) ) ;
#11352=CIRCLE ( 'NONE', #8407, 35.00000000000000000 ) ;
#11353=DIRECTION ( 'NONE',  ( 0.000000000000000000, -1.000000000000000000, -7.930164461608263644E-17 ) ) ;
#11356=EDGE_CURVE ( 'NONE', #10880, #3561, #508, .T. ) ;
#11360=ORIENTED_EDGE ( 'NONE', *, *, #11364, .T. ) ;
#11364=EDGE_CURVE ( 'NONE', #11808, #6290, #7067, .T. ) ;
#11368=AXIS2_PLACEMENT_3D ( 'NONE', #4586, #5243, #615 ) ;
#11377=PRODUCT_DEFINITION_SHAPE ( 'NONE', 'NONE',  #7149 ) ;
#11379=FACE_BOUND ( 'NONE', #5263, .T. ) ;
#11380=ORIENTED_EDGE ( 'NONE', *, *, #7228, .T. ) ;
#11394=EDGE_CURVE ( 'NONE', #1000, #3418, #12151, .T. ) ;
#11396=ORIENTED_EDGE ( 'NONE', *, *, #8809, .T. ) ;
#11398=VECTOR ( 'NONE', #4237, 1000.000000000000000 ) ;
#11404=DIRECTION ( 'NONE',  ( -0.000000000000000000, 1.000000000000000000, 7.930164461608263644E-17 ) ) ;
#11416=AXIS2_PLACEMENT_3D ( 'NONE', #5419, #4447, #1536 ) ;
#11429=DIRECTION ( 'NONE',  ( 0.000000000000000000, 0.000000000000000000, 1.000000000000000000 ) ) ;
#11431=CARTESIAN_POINT ( 'NONE',  ( -87.04832655144203102, 12.00000000000000000, -217.9289243767376831 ) ) ;
#11434=CARTESIAN_POINT ( 'NONE',  ( 6.247927005943220505E-13, -6.000000000000006217, -58.92135623730948879 ) ) ;
#11436=CARTESIAN_POINT ( 'NONE',  ( 1.562900236585165577E-12, -6.000000000000004441, 16.07864376269049700 ) ) ;
#11441=DIRECTION ( 'NONE',  ( -1.000000000000000000, -0.000000000000000000, -0.000000000000000000 ) ) ;
#11450=ADVANCED_FACE ( 'NONE', ( #5950 ), #5001, .F. ) ;
#11454=CARTESIAN_POINT ( 'NONE',  ( 35.00000000000000000, 12.00000000000001954, -124.6807709998040110 ) ) ;
#11458=EDGE_CURVE ( 'NONE', #3561, #1856, #8595, .T. ) ;
#11459=EDGE_CURVE ( 'NONE', #11527, #4090, #7800, .T. ) ;
#11460=DIRECTION ( 'NONE',  ( -0.000000000000000000, 1.000000000000000000, 7.930164461608263644E-17 ) ) ;
#11469=ORIENTED_EDGE ( 'NONE', *, *, #1462, .F. ) ;
#11470=EDGE_CURVE ( 'NONE', #7883, #5923, #8783, .T. ) ;
#11472=SHAPE_DEFINITION_REPRESENTATION ( #11377, #4488 ) ;
#11478=ADVANCED_FACE ( 'NONE', ( #10005 ), #4578, .F. ) ;
#11484=ORIENTED_EDGE ( 'NONE', *, *, #944, .F. ) ;
#11488=AXIS2_PLACEMENT_3D ( 'NONE', #8632, #3932, #148 ) ;
#11489=DIRECTION ( 'NONE',  ( 0.000000000000000000, -1.000000000000000000, -0.000000000000000000 ) ) ;
#11490=ORIENTED_EDGE ( 'NONE', *, *, #6855, .F. ) ;
#11493=CARTESIAN_POINT ( 'NONE',  ( 9.371890508914830252E-13, 12.00000000000000000, -36.42135623730949590 ) ) ;
#11498=AXIS2_PLACEMENT_3D ( 'NONE', #10692, #9889, #1422 ) ;
#11499=FACE_OUTER_BOUND ( 'NONE', #7366, .T. ) ;
#11501=FACE_BOUND ( 'NONE', #11072, .T. ) ;
#11507=CARTESIAN_POINT ( 'NONE',  ( 1.250503886288004501E-12, 0.000000000000000000, -13.92135623730950300 ) ) ;
#11515=CARTESIAN_POINT ( 'NONE',  ( 6.257111856936825515E-13, -6.000000000000004441, -73.92135623730949590 ) ) ;
#11516=DIRECTION ( 'NONE',  ( 0.000000000000000000, -1.000000000000000000, -7.930164461608263644E-17 ) ) ;
#11520=EDGE_CURVE ( 'NONE', #9670, #6223, #12047, .T. ) ;
#11525=ORIENTED_EDGE ( 'NONE', *, *, #1545, .F. ) ;
#11527=VERTEX_POINT ( 'NONE', #3626 ) ;
#11529=EDGE_LOOP ( 'NONE', ( #7416, #4049, #8910, #6488 ) ) ;
#11530=CARTESIAN_POINT ( 'NONE',  ( 1.562900236585165577E-12, 163.9999999999999716, 16.07864376269051121 ) ) ;
#11538=DIRECTION ( 'NONE',  ( 0.000000000000000000, 0.000000000000000000, 1.000000000000000000 ) ) ;
#11539=FACE_OUTER_BOUND ( 'NONE', #3517, .T. ) ;
#11543=CARTESIAN_POINT ( 'NONE',  ( 151.3258811035896656, 12.00000000000000000, -56.13263083939798292 ) ) ;
#11554=AXIS2_PLACEMENT_3D ( 'NONE', #10690, #2226, #9942 ) ;
#11555=DIRECTION ( 'NONE',  ( -0.000000000000000000, 1.000000000000000000, 7.930164461608263644E-17 ) ) ;
#11556=ORIENTED_EDGE ( 'NONE', *, *, #9846, .T. ) ;
#11565=EDGE_LOOP ( 'NONE', ( #1873, #4850 ) ) ;
#11568=DIRECTION ( 'NONE',  ( 0.000000000000000000, -0.000000000000000000, 1.000000000000000000 ) ) ;
#11574=CARTESIAN_POINT ( 'NONE',  ( -87.04832655144203102, 12.00000000000000000, -217.9289243767376831 ) ) ;
#11579=CYLINDRICAL_SURFACE ( 'NONE', #11778, 35.00000000000000000 ) ;
#11581=ORIENTED_EDGE ( 'NONE', *, *, #2840, .F. ) ;
#11590=EDGE_LOOP ( 'NONE', ( #122, #11141 ) ) ;
#11594=CARTESIAN_POINT ( 'NONE',  ( 1.249585401188644101E-12, 164.0000000000000000, -6.421356237309481685 ) ) ;
#11600=DIRECTION ( 'NONE',  ( -0.000000000000000000, 1.000000000000000000, 7.930164461608263644E-17 ) ) ;
#11602=EDGE_CURVE ( 'NONE', #11305, #7589, #906, .T. ) ;
#11606=ADVANCED_FACE ( 'NONE', ( #6239 ), #8290, .F. ) ;
#11607=ORIENTED_EDGE ( 'NONE', *, *, #3033, .T. ) ;
#11608=CARTESIAN_POINT ( 'NONE',  ( 9.371890508914830252E-13, 12.00000000000000000, -28.92135623730948524 ) ) ;
#11609=AXIS2_PLACEMENT_3D ( 'NONE', #7437, #2873, #7503 ) ;
#11610=EDGE_CURVE ( 'NONE', #5923, #7883, #2082, .T. ) ;
#11611=CARTESIAN_POINT ( 'NONE',  ( 144.0488662551573782, 12.00000000000000000, -146.9077238332702109 ) ) ;
#11614=EDGE_LOOP ( 'NONE', ( #5598, #85, #201, #810 ) ) ;
#11617=LINE ( 'NONE', #2210, #4961 ) ;
#11620=EDGE_CURVE ( 'NONE', #3812, #4792, #2459, .T. ) ;
#11624=DIRECTION ( 'NONE',  ( 0.000000000000000000, 0.000000000000000000, 1.000000000000000000 ) ) ;
#11626=VECTOR ( 'NONE', #854, 1000.000000000000000 ) ;
#11627=LINE ( 'NONE', #10681, #12160 ) ;
#11630=CIRCLE ( 'NONE', #10038, 7.500000000000007105 ) ;
#11631=FACE_OUTER_BOUND ( 'NONE', #10745, .T. ) ;
#11633=CARTESIAN_POINT ( 'NONE',  ( 1.387778780781445676E-14, -58.00000000000000711, 126.4213562373094959 ) ) ;
#11637=ORIENTED_EDGE ( 'NONE', *, *, #5332, .T. ) ;
#11643=LINE ( 'NONE', #8793, #10811 ) ;
#11649=ORIENTED_EDGE ( 'NONE', *, *, #7228, .F. ) ;
#11655=ADVANCED_FACE ( 'NONE', ( #11997 ), #7304, .F. ) ;
#11656=VERTEX_POINT ( 'NONE', #4458 ) ;
#11659=LINE ( 'NONE', #8633, #5615 ) ;
#11661=DIRECTION ( 'NONE',  ( 0.000000000000000000, 0.000000000000000000, 1.000000000000000000 ) ) ;
#11664=CARTESIAN_POINT ( 'NONE',  ( 2.186774452080127126E-12, 152.0000000000000000, 83.57864376269051832 ) ) ;
#11669=ADVANCED_FACE ( 'NONE', ( #8365 ), #5504, .F. ) ;
#11687=AXIS2_PLACEMENT_3D ( 'NONE', #3320, #2224, #7976 ) ;
#11689=DIRECTION ( 'NONE',  ( -0.000000000000000000, -1.000000000000000000, -0.000000000000000000 ) ) ;
#11691=ORIENTED_EDGE ( 'NONE', *, *, #1998, .F. ) ;
#11698=CARTESIAN_POINT ( 'NONE',  ( 2.187692937179487324E-12, 12.00000000000000000, 76.07864376269048989 ) ) ;
#11702=DIRECTION ( 'NONE',  ( 0.000000000000000000, 1.000000000000000000, 0.000000000000000000 ) ) ;
#11703=ORIENTED_EDGE ( 'NONE', *, *, #11161, .F. ) ;
#11705=ADVANCED_FACE ( 'NONE', ( #1673 ), #6250, .F. ) ;
#11706=AXIS2_PLACEMENT_3D ( 'NONE', #3611, #4627, #7580 ) ;
#11710=ORIENTED_EDGE ( 'NONE', *, *, #3820, .F. ) ;
#11713=ORIENTED_EDGE ( 'NONE', *, *, #7577, .T. ) ;
#11719=AXIS2_PLACEMENT_3D ( 'NONE', #1713, #8208, #10359 ) ;
#11731=FACE_OUTER_BOUND ( 'NONE', #11210, .T. ) ;
#11732=CYLINDRICAL_SURFACE ( 'NONE', #9706, 7.500000000000007105 ) ;
#11733=AXIS2_PLACEMENT_3D ( 'NONE', #1754, #9413, #6505 ) ;
#11734=ADVANCED_FACE ( 'NONE', ( #5432 ), #8237, .F. ) ;
#11737=DIRECTION ( 'NONE',  ( 0.000000000000000000, 0.000000000000000000, 1.000000000000000000 ) ) ;
#11744=DIRECTION ( 'NONE',  ( 0.000000000000000000, -1.000000000000000000, -7.930164461608263644E-17 ) ) ;
#11746=EDGE_CURVE ( 'NONE', #5383, #725, #2041, .T. ) ;
#11747=AXIS2_PLACEMENT_3D ( 'NONE', #10058, #11184, #12040 ) ;
#11748=AXIS2_PLACEMENT_3D ( 'NONE', #7750, #7511, #2813 ) ;
#11749=LINE ( 'NONE', #8888, #4177 ) ;
#11753=CIRCLE ( 'NONE', #5416, 7.500000000000007105 ) ;
#11754=AXIS2_PLACEMENT_3D ( 'NONE', #8835, #6920, #7793 ) ;
#11756=FACE_BOUND ( 'NONE', #12042, .T. ) ;
#11758=ADVANCED_FACE ( 'NONE', ( #2968 ), #5800, .F. ) ;
#11766=ORIENTED_EDGE ( 'NONE', *, *, #403, .T. ) ;
#11769=EDGE_CURVE ( 'NONE', #2477, #502, #4257, .T. ) ;
#11778=AXIS2_PLACEMENT_3D ( 'NONE', #2875, #3049, #77 ) ;
#11783=ORIENTED_EDGE ( 'NONE', *, *, #7123, .T. ) ;
#11788=AXIS2_PLACEMENT_3D ( 'NONE', #10421, #7459, #7520 ) ;
#11793=CIRCLE ( 'NONE', #1525, 7.500000000000007105 ) ;
#11796=FACE_BOUND ( 'NONE', #6265, .T. ) ;
#11807=ORIENTED_EDGE ( 'NONE', *, *, #6967, .T. ) ;
#11808=VERTEX_POINT ( 'NONE', #9403 ) ;
#11818=LINE ( 'NONE', #3333, #8851 ) ;
#11819=VERTEX_POINT ( 'NONE', #3771 ) ;
#11823=CIRCLE ( 'NONE', #7283, 7.500000000000007105 ) ;
#11824=ORIENTED_EDGE ( 'NONE', *, *, #7451, .F. ) ;
#11832=ORIENTED_EDGE ( 'NONE', *, *, #3485, .T. ) ;
#11847=ORIENTED_EDGE ( 'NONE', *, *, #9644, .T. ) ;
#11854=CARTESIAN_POINT ( 'NONE',  ( -45.53315400109751465, 12.00000000000000000, -230.3419396193594366 ) ) ;
#11860=FACE_OUTER_BOUND ( 'NONE', #7344, .T. ) ;
#11862=LINE ( 'NONE', #9763, #4602 ) ;
#11868=CARTESIAN_POINT ( 'NONE',  ( 1.875296586882326249E-12, -6.000000000000004441, 46.07864376269049700 ) ) ;
#11872=SURFACE_STYLE_USAGE ( .BOTH. , #3516 ) ;
#11883=DIRECTION ( 'NONE',  ( 0.000000000000000000, 0.000000000000000000, 1.000000000000000000 ) ) ;
#11885=ORIENTED_EDGE ( 'NONE', *, *, #5656, .T. ) ;
#11886=VERTEX_POINT ( 'NONE', #8033 ) ;
#11887=CIRCLE ( 'NONE', #5970, 7.500000000000007994 ) ;
#11889=CARTESIAN_POINT ( 'NONE',  ( 35.00000000000000000, 81.99999999999998579, 260.3192290001960032 ) ) ;
#11894=AXIS2_PLACEMENT_3D ( 'NONE', #900, #4668, #8446 ) ;
#11897=EDGE_CURVE ( 'NONE', #3398, #2733, #11627, .T. ) ;
#11899=DIRECTION ( 'NONE',  ( -0.000000000000000000, 1.000000000000000000, -0.000000000000000000 ) ) ;
#11904=CYLINDRICAL_SURFACE ( 'NONE', #1725, 7.500000000000013323 ) ;
#11910=AXIS2_PLACEMENT_3D ( 'NONE', #3764, #3948, #11429 ) ;
#11911=DIRECTION ( 'NONE',  ( 0.000000000000000000, -1.000000000000000000, -7.930164461608263644E-17 ) ) ;
#11914=EDGE_CURVE ( 'NONE', #4463, #647, #11948, .T. ) ;
#11915=VERTEX_POINT ( 'NONE', #1454 ) ;
#11919=CARTESIAN_POINT ( 'NONE',  ( 3.123963502971610252E-13, 0.000000000000000000, -88.92135623730948168 ) ) ;
#11921=VECTOR ( 'NONE', #723, 1000.000000000000000 ) ;
#11928=DIRECTION ( 'NONE',  ( -0.000000000000000000, -1.000000000000000000, -0.000000000000000000 ) ) ;
#11932=CYLINDRICAL_SURFACE ( 'NONE', #9563, 7.500000000000007105 ) ;
#11934=DIRECTION ( 'NONE',  ( -1.000000000000000000, -0.000000000000000000, 0.000000000000000000 ) ) ;
#11947=VERTEX_POINT ( 'NONE', #3417 ) ;
#11948=CIRCLE ( 'NONE', #1691, 7.500000000000007105 ) ;
#11950=ADVANCED_FACE ( 'NONE', ( #5338 ), #3304, .F. ) ;
#11955=LINE ( 'NONE', #7441, #133 ) ;
#11957=AXIS2_PLACEMENT_3D ( 'NONE', #9048, #10904, #7955 ) ;
#11959=CARTESIAN_POINT ( 'NONE',  ( 1.874378101782966050E-12, 152.0000000000000000, 61.07864376269052542 ) ) ;
#11960=DIRECTION ( 'NONE',  ( 0.000000000000000000, 1.000000000000000000, 0.000000000000000000 ) ) ;
#11967=CARTESIAN_POINT ( 'NONE',  ( 6.257111856936825515E-13, 12.00000000000000000, -73.92135623730949590 ) ) ;
#11971=EDGE_CURVE ( 'NONE', #2282, #6215, #6815, .T. ) ;
#11972=DIRECTION ( 'NONE',  ( -0.000000000000000000, 1.000000000000000000, 0.000000000000000000 ) ) ;
#11979=ORIENTED_EDGE ( 'NONE', *, *, #8508, .F. ) ;
#11988=EDGE_CURVE ( 'NONE', #8074, #8885, #1578, .T. ) ;
#11989=VERTEX_POINT ( 'NONE', #7206 ) ;
#11991=DIRECTION ( 'NONE',  ( -0.000000000000000000, 1.000000000000000000, -0.000000000000000000 ) ) ;
#11997=FACE_OUTER_BOUND ( 'NONE', #753, .T. ) ;
#11998=VERTEX_POINT ( 'NONE', #9986 ) ;
#12004=AXIS2_PLACEMENT_3D ( 'NONE', #1431, #9896, #3388 ) ;
#12014=DIRECTION ( 'NONE',  ( 0.000000000000000000, 1.000000000000000000, 0.000000000000000000 ) ) ;
#12015=CARTESIAN_POINT ( 'NONE',  ( 1.249585401188644101E-12, 0.000000000000000000, -6.421356237309494119 ) ) ;
#12016=CIRCLE ( 'NONE', #3521, 7.500000000000007105 ) ;
#12036=EDGE_CURVE ( 'NONE', #10023, #3744, #2468, .T. ) ;
#12038=DIRECTION ( 'NONE',  ( 0.000000000000000000, -1.000000000000000000, -7.930164461608263644E-17 ) ) ;
#12040=DIRECTION ( 'NONE',  ( 0.000000000000000000, 0.000000000000000000, -1.000000000000000000 ) ) ;
#12042=EDGE_LOOP ( 'NONE', ( #9593, #10156 ) ) ;
#12045=CARTESIAN_POINT ( 'NONE',  ( 9.381075359908434252E-13, 12.00000000000000000, -43.92135623730950300 ) ) ;
#12046=CYLINDRICAL_SURFACE ( 'NONE', #2337, 7.500000000000020428 ) ;
#12047=LINE ( 'NONE', #7226, #1887 ) ;
#12050=ORIENTED_EDGE ( 'NONE', *, *, #1943, .T. ) ;
#12052=LINE ( 'NONE', #6612, #175 ) ;
#12053=CARTESIAN_POINT ( 'NONE',  ( 6.247927005943220505E-13, 12.00000000000000000, -66.42135623730949590 ) ) ;
#12060=ORIENTED_EDGE ( 'NONE', *, *, #11988, .F. ) ;
#12061=DIRECTION ( 'NONE',  ( -0.000000000000000000, 1.000000000000000000, 0.000000000000000000 ) ) ;
#12072=ORIENTED_EDGE ( 'NONE', *, *, #9179, .T. ) ;
#12083=LINE ( 'NONE', #11087, #6418 ) ;
#12084=AXIS2_PLACEMENT_3D ( 'NONE', #6979, #3149, #1304 ) ;
#12093=DIRECTION ( 'NONE',  ( -0.000000000000000000, 1.000000000000000000, 7.930164461608263644E-17 ) ) ;
#12096=CARTESIAN_POINT ( 'NONE',  ( -126.4213562373094959, 0.000000000000000000, -7.499999999999991118 ) ) ;
#12099=LINE ( 'NONE', #10977, #2940 ) ;
#12105=CARTESIAN_POINT ( 'NONE',  ( 2.186774452080127126E-12, 163.9999999999999716, 83.57864376269051832 ) ) ;
#12107=ORIENTED_EDGE ( 'NONE', *, *, #2857, .T. ) ;
#12108=DIRECTION ( 'NONE',  ( 0.000000000000000000, 0.000000000000000000, 1.000000000000000000 ) ) ;
#12114=DIRECTION ( 'NONE',  ( 0.000000000000000000, 1.000000000000000000, 0.000000000000000000 ) ) ;
#12119=VERTEX_POINT ( 'NONE', #584 ) ;
#12128=DIRECTION ( 'NONE',  ( 0.000000000000000000, 0.000000000000000000, 1.000000000000000000 ) ) ;
#12131=AXIS2_PLACEMENT_3D ( 'NONE', #9691, #10440, #7909 ) ;
#12137=ADVANCED_FACE ( 'NONE', ( #4950 ), #3268, .F. ) ;
#12138=ORIENTED_EDGE ( 'NONE', *, *, #5532, .F. ) ;
#12141=AXIS2_PLACEMENT_3D ( 'NONE', #11594, #7884, #3226 ) ;
#12146=FACE_OUTER_BOUND ( 'NONE', #11004, .T. ) ;
#12151=CIRCLE ( 'NONE', #5029, 134.9999999999999716 ) ;
#12153=CYLINDRICAL_SURFACE ( 'NONE', #2908, 7.500000000000007105 ) ;
#12157=DIRECTION ( 'NONE',  ( -1.000000000000000000, -0.000000000000000000, 0.000000000000000000 ) ) ;
#12160=VECTOR ( 'NONE', #2219, 1000.000000000000000 ) ;
#12162=DIRECTION ( 'NONE',  ( 0.000000000000000000, -1.000000000000000000, -7.930164461608263644E-17 ) ) ;
#12182=FACE_OUTER_BOUND ( 'NONE', #3654, .T. ) ;
#12187=CIRCLE ( 'NONE', #5061, 7.500000000000007105 ) ;
#12207=EDGE_LOOP ( 'NONE', ( #193, #7396, #1223, #1636 ) ) ;
#12208=AXIS2_PLACEMENT_3D ( 'NONE', #3499, #11054, #6179 ) ;
#12209=EDGE_CURVE ( 'NONE', #918, #1702, #6185, .T. ) ;
#12216=ORIENTED_EDGE ( 'NONE', *, *, #9101, .F. ) ;
#12217=AXIS2_PLACEMENT_3D ( 'NONE', #8849, #11702, #3217 ) ;
#12218=FACE_BOUND ( 'NONE', #6760, .T. ) ;
#12227=VECTOR ( 'NONE', #3711, 1000.000000000000000 ) ;
#12228=EDGE_CURVE ( 'NONE', #4052, #1330, #4466, .T. ) ;
#12233=CARTESIAN_POINT ( 'NONE',  ( 9.371890508914830252E-13, 0.000000000000000000, -28.92135623730948524 ) ) ;
ENDSEC;
END-ISO-10303-21;
